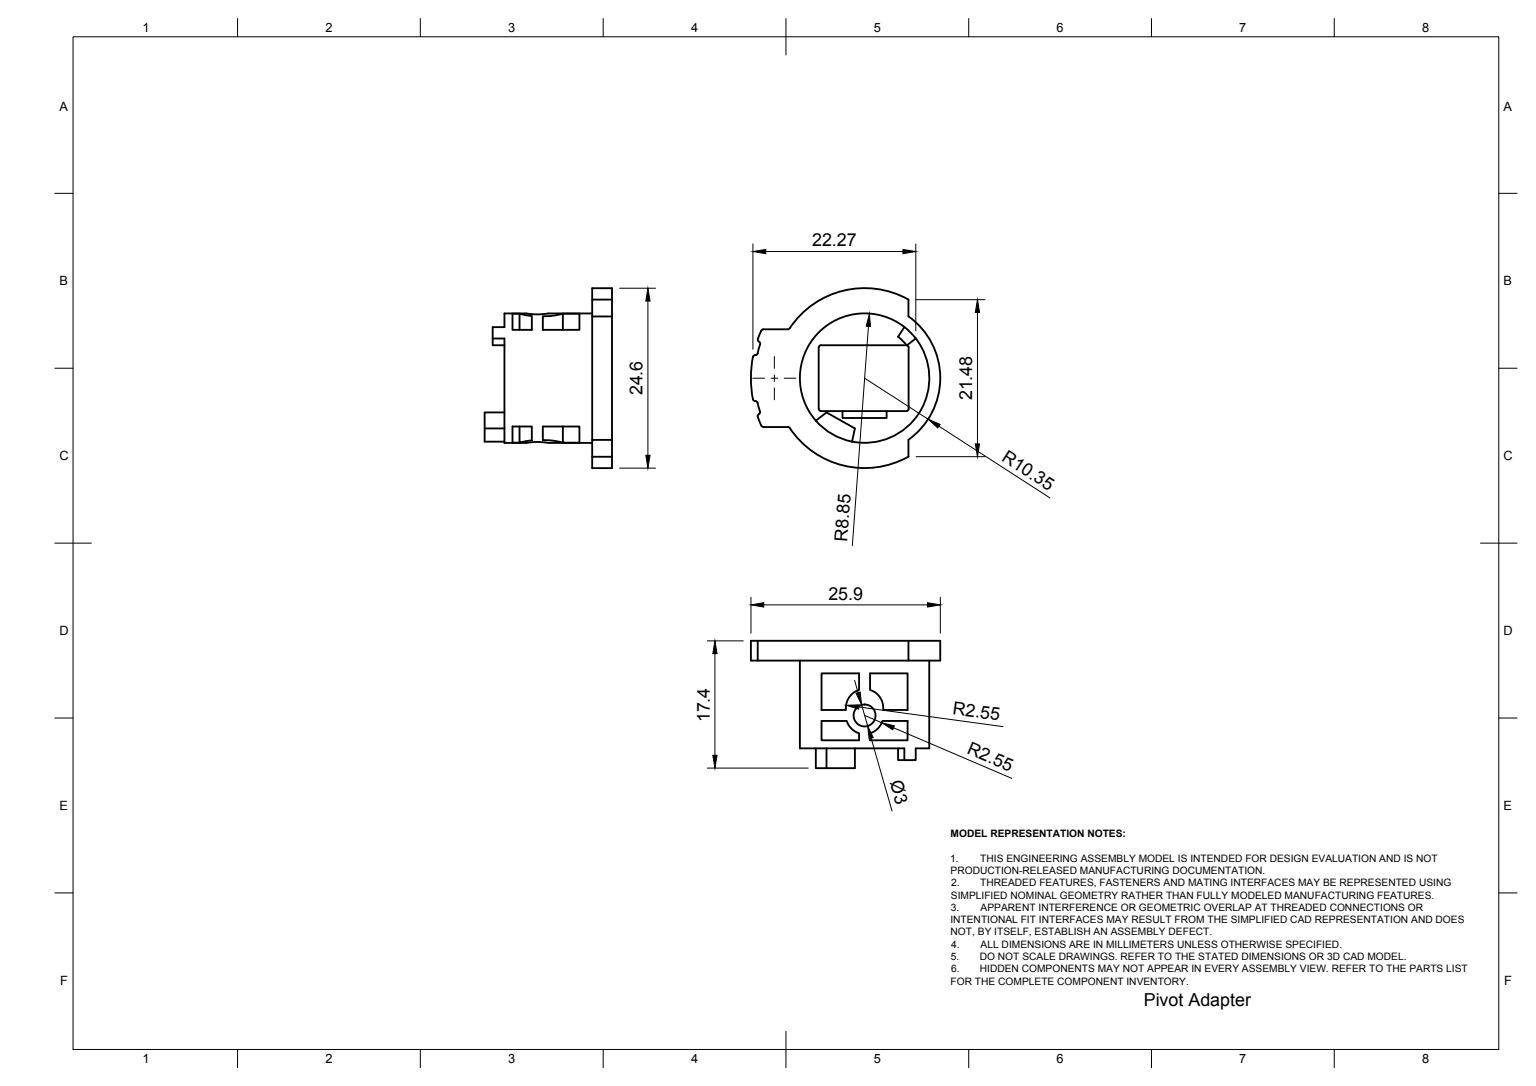
ISO-10303-21;
HEADER;
/* Generated by software containing ST-Developer
 * from STEP Tools, Inc. (www.steptools.com) 
 */

FILE_DESCRIPTION(
/* description */ ('STEP AP214'),
/* implementation_level */ '2;1');

FILE_NAME(
/* name */ 'Pivot Adapter.step',
/* time_stamp */ '2026-10-06T00:19:40-07:00',
/* author */ (''),
/* organization */ (''),
/* preprocessor_version */ 'ST-DEVELOPER v20.2',
/* originating_system */ 'Autodesk Translation Framework v15.15.0.0',
/* authorisation */ '');

FILE_SCHEMA (('AUTOMOTIVE_DESIGN { 1 0 10303 214 3 1 1 }'));
ENDSEC;

DATA;
#10=MECHANICAL_DESIGN_GEOMETRIC_PRESENTATION_REPRESENTATION('',(#2072),#98302);
#443=TOROIDAL_SURFACE('',#38348,4.64715395326,0.3);
#444=TOROIDAL_SURFACE('',#38570,0.6,0.3);
#445=TOROIDAL_SURFACE('',#38577,0.6,0.3);
#446=TOROIDAL_SURFACE('',#38588,0.6,0.3);
#447=TOROIDAL_SURFACE('',#38591,4.47840533247,0.3);
#448=TOROIDAL_SURFACE('',#38598,0.6,0.3);
#859=SPHERICAL_SURFACE('',#38392,4.49);
#860=SPHERICAL_SURFACE('',#38586,0.3);
#861=SPHERICAL_SURFACE('',#38596,0.3);
#1252=B_SPLINE_SURFACE_WITH_KNOTS('',5,5,((#98145,#98146,#98147,#98148,
#98149,#98150),(#98151,#98152,#98153,#98154,#98155,#98156),(#98157,#98158,
#98159,#98160,#98161,#98162),(#98163,#98164,#98165,#98166,#98167,#98168),
(#98169,#98170,#98171,#98172,#98173,#98174),(#98175,#98176,#98177,#98178,
#98179,#98180)),.UNSPECIFIED.,.F.,.F.,.F.,(6,6),(6,6),(2.82953519577,3.40560970652),
(0.,0.3),.UNSPECIFIED.);
#1253=B_SPLINE_SURFACE_WITH_KNOTS('',5,5,((#98207,#98208,#98209,#98210,
#98211,#98212),(#98213,#98214,#98215,#98216,#98217,#98218),(#98219,#98220,
#98221,#98222,#98223,#98224),(#98225,#98226,#98227,#98228,#98229,#98230),
(#98231,#98232,#98233,#98234,#98235,#98236),(#98237,#98238,#98239,#98240,
#98241,#98242)),.UNSPECIFIED.,.F.,.F.,.F.,(6,6),(6,6),(4.13551351914,4.71167786523),
(0.,0.3),.UNSPECIFIED.);
#1316=FACE_BOUND('',#7509,.T.);
#1317=FACE_BOUND('',#7564,.T.);
#1318=FACE_BOUND('',#7565,.T.);
#1319=FACE_BOUND('',#7599,.T.);
#1320=FACE_BOUND('',#7600,.T.);
#1321=FACE_BOUND('',#7601,.T.);
#1322=FACE_BOUND('',#7602,.T.);
#1323=FACE_BOUND('',#7603,.T.);
#1324=FACE_BOUND('',#7604,.T.);
#1325=FACE_BOUND('',#7605,.T.);
#1326=FACE_BOUND('',#7606,.T.);
#1327=FACE_BOUND('',#7607,.T.);
#1328=FACE_BOUND('',#7608,.T.);
#1329=FACE_BOUND('',#7619,.T.);
#1330=FACE_BOUND('',#7631,.T.);
#1331=FACE_BOUND('',#7634,.T.);
#2027=B_SPLINE_CURVE_WITH_KNOTS('',3,(#97465,#97466,#97467,#97468,#97469,
#97470,#97471),.UNSPECIFIED.,.F.,.F.,(4,3,4),(-4.71167786523,-4.28310422559678,
-4.13551354843282),.UNSPECIFIED.);
#2028=B_SPLINE_CURVE_WITH_KNOTS('',5,(#97472,#97473,#97474,#97475,#97476,
#97477),.UNSPECIFIED.,.F.,.F.,(6,6),(-3.40560970652,-2.82953519577),
 .UNSPECIFIED.);
#2029=B_SPLINE_CURVE_WITH_KNOTS('',3,(#97520,#97521,#97522,#97523,#97524,
#97525,#97526,#97527,#97528,#97529,#97530,#97531,#97532,#97533),
 .UNSPECIFIED.,.F.,.F.,(4,2,2,2,2,2,4),(0.22648251624436,0.28310233584346,
0.33972215544256,0.39634359396564,0.452965032488721,0.509586471011801,0.566207909534882),
 .UNSPECIFIED.);
#2030=B_SPLINE_CURVE_WITH_KNOTS('',3,(#97534,#97535,#97536,#97537,#97538,
#97539,#97540,#97541,#97542,#97543,#97544,#97545,#97546,#97547,#97548,#97549,
#97550,#97551,#97552,#97553,#97554,#97555,#97556),.UNSPECIFIED.,.F.,.F.,
(4,2,2,2,2,2,3,2,2,2,4),(0.566207909534882,0.622827729133982,0.679447548733081,
0.736067368332181,0.792687187931281,0.849308626454361,0.905930064977442,
0.962551503500522,1.0191729420236,1.0757927616227,1.1324125812218),
 .UNSPECIFIED.);
#2031=B_SPLINE_CURVE_WITH_KNOTS('',3,(#97583,#97584,#97585,#97586,#97587,
#97588,#97589,#97590,#97591,#97592),.UNSPECIFIED.,.F.,.F.,(4,2,2,2,4),(1.23339450152361,
1.25641237692672,1.35304825225328,1.44970846052674,1.5463686688002),
 .UNSPECIFIED.);
#2032=B_SPLINE_CURVE_WITH_KNOTS('',3,(#97622,#97623,#97624,#97625,#97626,
#97627,#97628,#97629,#97630,#97631),.UNSPECIFIED.,.F.,.F.,(4,2,2,2,4),(0.0736329241578598,
0.0966612073704035,0.193322414740807,0.289959287879085,0.312978165630601),
 .UNSPECIFIED.);
#2033=B_SPLINE_CURVE_WITH_KNOTS('',3,(#97652,#97653,#97654,#97655,#97656,
#97657,#97658,#97659,#97660,#97661),.UNSPECIFIED.,.F.,.F.,(4,2,2,2,4),(-0.699559397876643,
-0.676531114664321,-0.579869907293917,-0.48323303415564,-0.460214156403763),
 .UNSPECIFIED.);
#2034=B_SPLINE_CURVE_WITH_KNOTS('',3,(#97691,#97692,#97693,#97694,#97695,
#97696,#97697,#97698,#97699,#97700),.UNSPECIFIED.,.F.,.F.,(4,2,2,2,4),(0.773184334400102,
0.869844542673565,0.966504750947028,1.06314062627359,1.08615850163623),
 .UNSPECIFIED.);
#2035=B_SPLINE_CURVE_WITH_KNOTS('',3,(#97759,#97760,#97761,#97762,#97763,
#97764),.UNSPECIFIED.,.F.,.F.,(4,2,4),(0.566207909534882,0.622827729133982,
0.679447548733081),.UNSPECIFIED.);
#2036=B_SPLINE_CURVE_WITH_KNOTS('',3,(#97765,#97766,#97767,#97768,#97769,
#97770,#97771,#97772,#97773,#97774,#97775,#97776,#97777,#97778,#97779,#97780,
#97781,#97782,#97783,#97784,#97785,#97786,#97787,#97788,#97789,#97790,#97791,
#97792,#97793,#97794,#97795),.UNSPECIFIED.,.F.,.F.,(4,2,2,2,3,2,2,2,2,2,
2,2,2,2,4),(-0.22648251624436,-0.169862696645261,-0.113242877046161,-0.0566214385230804,
0.,0.0566214385230803,0.113242877046161,0.169862696645261,0.22648251624436,
0.28310233584346,0.33972215544256,0.39634359396564,0.452965032488721,0.509586471011801,
0.566207909534882),.UNSPECIFIED.);
#2037=B_SPLINE_CURVE_WITH_KNOTS('',3,(#97811,#97812,#97813,#97814,#97815,
#97816,#97817,#97818,#97819,#97820),.UNSPECIFIED.,.F.,.F.,(4,2,2,2,4),(-0.312974167276592,
-0.289956291873489,-0.193320416546926,-0.0966602082734631,0.),
 .UNSPECIFIED.);
#2038=B_SPLINE_CURVE_WITH_KNOTS('',3,(#97841,#97842,#97843,#97844,#97845,
#97846,#97847,#97848,#97849,#97850),.UNSPECIFIED.,.F.,.F.,(4,2,2,2,4),(-0.773184334400102,
-0.676524126126639,-0.579863917853176,-0.483228042526613,-0.460210167163969),
 .UNSPECIFIED.);
#2039=B_SPLINE_CURVE_WITH_KNOTS('',3,(#97873,#97874,#97875,#97876,#97877,
#97878,#97879,#97880,#97881,#97882),.UNSPECIFIED.,.F.,.F.,(4,2,2,2,4),(0.846825246192806,
0.869853529405128,0.966514736775532,1.06315160991381,1.08617048766569),
 .UNSPECIFIED.);
#2040=B_SPLINE_CURVE_WITH_KNOTS('',3,(#97903,#97904,#97905,#97906,#97907,
#97908,#97909,#97910,#97911,#97912),.UNSPECIFIED.,.F.,.F.,(4,2,2,2,4),(-1.47275171991159,
-1.44972343669905,-1.35306222932864,-1.25642535619036,-1.23340647843885),
 .UNSPECIFIED.);
#2041=B_SPLINE_CURVE_WITH_KNOTS('',3,(#98184,#98185,#98186,#98187,#98188,
#98189,#98190,#98191,#98192,#98193),.UNSPECIFIED.,.F.,.F.,(4,3,3,4),(-3.40560970652,
-3.15933845109684,-2.86373280280867,-2.82953519577),.UNSPECIFIED.);
#2042=B_SPLINE_CURVE_WITH_KNOTS('',3,(#98244,#98245,#98246,#98247,#98248,
#98249,#98250),.UNSPECIFIED.,.F.,.F.,(4,3,4),(-4.71167786523,-4.23171687797706,
-4.13551351914),.UNSPECIFIED.);
#2052=SHAPE_REPRESENTATION_RELATIONSHIP('SRR','None',#98349,#2062);
#2062=ADVANCED_BREP_SHAPE_REPRESENTATION('',(#2081),#98301);
#2072=STYLED_ITEM('',(#98399),#2081);
#2081=MANIFOLD_SOLID_BREP('Body1',#34178);
#2452=PLANE('',#38355);
#2453=PLANE('',#38358);
#2454=PLANE('',#38359);
#2455=PLANE('',#38362);
#2456=PLANE('',#38363);
#2457=PLANE('',#38365);
#2458=PLANE('',#38366);
#2459=PLANE('',#38367);
#2460=PLANE('',#38368);
#2461=PLANE('',#38372);
#2462=PLANE('',#38394);
#2463=PLANE('',#38402);
#2464=PLANE('',#38405);
#2465=PLANE('',#38407);
#2466=PLANE('',#38409);
#2467=PLANE('',#38411);
#2468=PLANE('',#38412);
#2469=PLANE('',#38414);
#2470=PLANE('',#38416);
#2471=PLANE('',#38418);
#2472=PLANE('',#38420);
#2473=PLANE('',#38422);
#2474=PLANE('',#38424);
#2475=PLANE('',#38427);
#2476=PLANE('',#38428);
#2477=PLANE('',#38430);
#2478=PLANE('',#38432);
#2479=PLANE('',#38434);
#2480=PLANE('',#38436);
#2481=PLANE('',#38437);
#2482=PLANE('',#38439);
#2483=PLANE('',#38441);
#2484=PLANE('',#38445);
#2485=PLANE('',#38449);
#2486=PLANE('',#38450);
#2487=PLANE('',#38455);
#2488=PLANE('',#38460);
#2489=PLANE('',#38462);
#2490=PLANE('',#38465);
#2491=PLANE('',#38466);
#2492=PLANE('',#38469);
#2493=PLANE('',#38470);
#2494=PLANE('',#38472);
#2495=PLANE('',#38476);
#2496=PLANE('',#38477);
#2497=PLANE('',#38481);
#2498=PLANE('',#38485);
#2499=PLANE('',#38512);
#2500=PLANE('',#38515);
#2501=PLANE('',#38520);
#2502=PLANE('',#38533);
#2503=PLANE('',#38540);
#2504=PLANE('',#38553);
#2505=PLANE('',#38556);
#2506=PLANE('',#38558);
#2507=PLANE('',#38559);
#2508=PLANE('',#38560);
#2509=PLANE('',#38562);
#2510=PLANE('',#38564);
#2511=PLANE('',#38568);
#2512=PLANE('',#38569);
#2513=PLANE('',#38576);
#2514=PLANE('',#38583);
#2515=PLANE('',#38594);
#2516=PLANE('',#38601);
#2517=PLANE('',#38602);
#2518=PLANE('',#38603);
#2519=PLANE('',#38604);
#2520=PLANE('',#38605);
#3234=CYLINDRICAL_SURFACE('',#38360,7.28184557105);
#3235=CYLINDRICAL_SURFACE('',#38370,1.2046272227);
#3236=CYLINDRICAL_SURFACE('',#38403,1.5);
#3237=CYLINDRICAL_SURFACE('',#38410,2.54997399005);
#3238=CYLINDRICAL_SURFACE('',#38419,2.55);
#3239=CYLINDRICAL_SURFACE('',#38426,2.55);
#3240=CYLINDRICAL_SURFACE('',#38435,2.54997399005);
#3241=CYLINDRICAL_SURFACE('',#38443,7.35);
#3242=CYLINDRICAL_SURFACE('',#38444,7.35);
#3243=CYLINDRICAL_SURFACE('',#38451,8.85);
#3244=CYLINDRICAL_SURFACE('',#38453,1.8);
#3245=CYLINDRICAL_SURFACE('',#38456,1.8);
#3246=CYLINDRICAL_SURFACE('',#38458,1.5);
#3247=CYLINDRICAL_SURFACE('',#38463,2.54997399005);
#3248=CYLINDRICAL_SURFACE('',#38467,2.54997399005);
#3249=CYLINDRICAL_SURFACE('',#38474,2.55);
#3250=CYLINDRICAL_SURFACE('',#38479,2.55);
#3251=CYLINDRICAL_SURFACE('',#38482,0.3);
#3252=CYLINDRICAL_SURFACE('',#38510,12.3);
#3253=CYLINDRICAL_SURFACE('',#38513,10.35);
#3254=CYLINDRICAL_SURFACE('',#38516,12.3);
#3255=CYLINDRICAL_SURFACE('',#38518,0.3);
#3256=CYLINDRICAL_SURFACE('',#38521,0.3);
#3257=CYLINDRICAL_SURFACE('',#38523,15.55);
#3258=CYLINDRICAL_SURFACE('',#38525,0.3);
#3259=CYLINDRICAL_SURFACE('',#38527,0.299999999999999);
#3260=CYLINDRICAL_SURFACE('',#38529,15.0204936174);
#3261=CYLINDRICAL_SURFACE('',#38531,0.3);
#3262=CYLINDRICAL_SURFACE('',#38534,0.3);
#3263=CYLINDRICAL_SURFACE('',#38536,15.55);
#3264=CYLINDRICAL_SURFACE('',#38538,0.3);
#3265=CYLINDRICAL_SURFACE('',#38541,0.3);
#3266=CYLINDRICAL_SURFACE('',#38543,15.0204936174);
#3267=CYLINDRICAL_SURFACE('',#38545,0.3);
#3268=CYLINDRICAL_SURFACE('',#38547,0.3);
#3269=CYLINDRICAL_SURFACE('',#38549,15.55);
#3270=CYLINDRICAL_SURFACE('',#38551,0.3);
#3271=CYLINDRICAL_SURFACE('',#38554,0.3);
#3272=CYLINDRICAL_SURFACE('',#38565,8.85);
#3273=CYLINDRICAL_SURFACE('',#38573,0.3);
#3274=CYLINDRICAL_SURFACE('',#38574,0.3);
#3275=CYLINDRICAL_SURFACE('',#38580,0.3);
#3276=CYLINDRICAL_SURFACE('',#38581,0.300000000000002);
#3277=CYLINDRICAL_SURFACE('',#38590,0.3);
#3278=CYLINDRICAL_SURFACE('',#38600,0.3);
#5294=FACE_OUTER_BOUND('',#7496,.T.);
#5295=FACE_OUTER_BOUND('',#7497,.T.);
#5296=FACE_OUTER_BOUND('',#7498,.T.);
#5297=FACE_OUTER_BOUND('',#7499,.T.);
#5298=FACE_OUTER_BOUND('',#7500,.T.);
#5299=FACE_OUTER_BOUND('',#7501,.T.);
#5300=FACE_OUTER_BOUND('',#7502,.T.);
#5301=FACE_OUTER_BOUND('',#7503,.T.);
#5302=FACE_OUTER_BOUND('',#7504,.T.);
#5303=FACE_OUTER_BOUND('',#7505,.T.);
#5304=FACE_OUTER_BOUND('',#7506,.T.);
#5305=FACE_OUTER_BOUND('',#7507,.T.);
#5306=FACE_OUTER_BOUND('',#7508,.T.);
#5307=FACE_OUTER_BOUND('',#7510,.T.);
#5308=FACE_OUTER_BOUND('',#7511,.T.);
#5309=FACE_OUTER_BOUND('',#7512,.T.);
#5310=FACE_OUTER_BOUND('',#7513,.T.);
#5311=FACE_OUTER_BOUND('',#7514,.T.);
#5312=FACE_OUTER_BOUND('',#7515,.T.);
#5313=FACE_OUTER_BOUND('',#7516,.T.);
#5314=FACE_OUTER_BOUND('',#7517,.T.);
#5315=FACE_OUTER_BOUND('',#7518,.T.);
#5316=FACE_OUTER_BOUND('',#7519,.T.);
#5317=FACE_OUTER_BOUND('',#7520,.T.);
#5318=FACE_OUTER_BOUND('',#7521,.T.);
#5319=FACE_OUTER_BOUND('',#7522,.T.);
#5320=FACE_OUTER_BOUND('',#7523,.T.);
#5321=FACE_OUTER_BOUND('',#7524,.T.);
#5322=FACE_OUTER_BOUND('',#7525,.T.);
#5323=FACE_OUTER_BOUND('',#7526,.T.);
#5324=FACE_OUTER_BOUND('',#7527,.T.);
#5325=FACE_OUTER_BOUND('',#7528,.T.);
#5326=FACE_OUTER_BOUND('',#7529,.T.);
#5327=FACE_OUTER_BOUND('',#7530,.T.);
#5328=FACE_OUTER_BOUND('',#7531,.T.);
#5329=FACE_OUTER_BOUND('',#7532,.T.);
#5330=FACE_OUTER_BOUND('',#7533,.T.);
#5331=FACE_OUTER_BOUND('',#7534,.T.);
#5332=FACE_OUTER_BOUND('',#7535,.T.);
#5333=FACE_OUTER_BOUND('',#7536,.T.);
#5334=FACE_OUTER_BOUND('',#7537,.T.);
#5335=FACE_OUTER_BOUND('',#7538,.T.);
#5336=FACE_OUTER_BOUND('',#7539,.T.);
#5337=FACE_OUTER_BOUND('',#7540,.T.);
#5338=FACE_OUTER_BOUND('',#7541,.T.);
#5339=FACE_OUTER_BOUND('',#7542,.T.);
#5340=FACE_OUTER_BOUND('',#7543,.T.);
#5341=FACE_OUTER_BOUND('',#7544,.T.);
#5342=FACE_OUTER_BOUND('',#7545,.T.);
#5343=FACE_OUTER_BOUND('',#7546,.T.);
#5344=FACE_OUTER_BOUND('',#7547,.T.);
#5345=FACE_OUTER_BOUND('',#7548,.T.);
#5346=FACE_OUTER_BOUND('',#7549,.T.);
#5347=FACE_OUTER_BOUND('',#7550,.T.);
#5348=FACE_OUTER_BOUND('',#7551,.T.);
#5349=FACE_OUTER_BOUND('',#7552,.T.);
#5350=FACE_OUTER_BOUND('',#7553,.T.);
#5351=FACE_OUTER_BOUND('',#7554,.T.);
#5352=FACE_OUTER_BOUND('',#7555,.T.);
#5353=FACE_OUTER_BOUND('',#7556,.T.);
#5354=FACE_OUTER_BOUND('',#7557,.T.);
#5355=FACE_OUTER_BOUND('',#7558,.T.);
#5356=FACE_OUTER_BOUND('',#7559,.T.);
#5357=FACE_OUTER_BOUND('',#7560,.T.);
#5358=FACE_OUTER_BOUND('',#7561,.T.);
#5359=FACE_OUTER_BOUND('',#7562,.T.);
#5360=FACE_OUTER_BOUND('',#7563,.T.);
#5361=FACE_OUTER_BOUND('',#7566,.T.);
#5362=FACE_OUTER_BOUND('',#7567,.T.);
#5363=FACE_OUTER_BOUND('',#7568,.T.);
#5364=FACE_OUTER_BOUND('',#7569,.T.);
#5365=FACE_OUTER_BOUND('',#7570,.T.);
#5366=FACE_OUTER_BOUND('',#7571,.T.);
#5367=FACE_OUTER_BOUND('',#7572,.T.);
#5368=FACE_OUTER_BOUND('',#7573,.T.);
#5369=FACE_OUTER_BOUND('',#7574,.T.);
#5370=FACE_OUTER_BOUND('',#7575,.T.);
#5371=FACE_OUTER_BOUND('',#7576,.T.);
#5372=FACE_OUTER_BOUND('',#7577,.T.);
#5373=FACE_OUTER_BOUND('',#7578,.T.);
#5374=FACE_OUTER_BOUND('',#7579,.T.);
#5375=FACE_OUTER_BOUND('',#7580,.T.);
#5376=FACE_OUTER_BOUND('',#7581,.T.);
#5377=FACE_OUTER_BOUND('',#7582,.T.);
#5378=FACE_OUTER_BOUND('',#7583,.T.);
#5379=FACE_OUTER_BOUND('',#7584,.T.);
#5380=FACE_OUTER_BOUND('',#7585,.T.);
#5381=FACE_OUTER_BOUND('',#7586,.T.);
#5382=FACE_OUTER_BOUND('',#7587,.T.);
#5383=FACE_OUTER_BOUND('',#7588,.T.);
#5384=FACE_OUTER_BOUND('',#7589,.T.);
#5385=FACE_OUTER_BOUND('',#7590,.T.);
#5386=FACE_OUTER_BOUND('',#7591,.T.);
#5387=FACE_OUTER_BOUND('',#7592,.T.);
#5388=FACE_OUTER_BOUND('',#7593,.T.);
#5389=FACE_OUTER_BOUND('',#7594,.T.);
#5390=FACE_OUTER_BOUND('',#7595,.T.);
#5391=FACE_OUTER_BOUND('',#7596,.T.);
#5392=FACE_OUTER_BOUND('',#7597,.T.);
#5393=FACE_OUTER_BOUND('',#7598,.T.);
#5394=FACE_OUTER_BOUND('',#7609,.T.);
#5395=FACE_OUTER_BOUND('',#7610,.T.);
#5396=FACE_OUTER_BOUND('',#7611,.T.);
#5397=FACE_OUTER_BOUND('',#7612,.T.);
#5398=FACE_OUTER_BOUND('',#7613,.T.);
#5399=FACE_OUTER_BOUND('',#7614,.T.);
#5400=FACE_OUTER_BOUND('',#7615,.T.);
#5401=FACE_OUTER_BOUND('',#7616,.T.);
#5402=FACE_OUTER_BOUND('',#7617,.T.);
#5403=FACE_OUTER_BOUND('',#7618,.T.);
#5404=FACE_OUTER_BOUND('',#7620,.T.);
#5405=FACE_OUTER_BOUND('',#7621,.T.);
#5406=FACE_OUTER_BOUND('',#7622,.T.);
#5407=FACE_OUTER_BOUND('',#7623,.T.);
#5408=FACE_OUTER_BOUND('',#7624,.T.);
#5409=FACE_OUTER_BOUND('',#7625,.T.);
#5410=FACE_OUTER_BOUND('',#7626,.T.);
#5411=FACE_OUTER_BOUND('',#7627,.T.);
#5412=FACE_OUTER_BOUND('',#7628,.T.);
#5413=FACE_OUTER_BOUND('',#7629,.T.);
#5414=FACE_OUTER_BOUND('',#7630,.T.);
#5415=FACE_OUTER_BOUND('',#7632,.T.);
#5416=FACE_OUTER_BOUND('',#7633,.T.);
#5417=FACE_OUTER_BOUND('',#7635,.T.);
#5418=FACE_OUTER_BOUND('',#7636,.T.);
#7496=EDGE_LOOP('',(#31335,#31336,#31337,#31338,#31339,#31340));
#7497=EDGE_LOOP('',(#31341,#31342,#31343,#31344,#31345));
#7498=EDGE_LOOP('',(#31346,#31347,#31348,#31349));
#7499=EDGE_LOOP('',(#31350,#31351,#31352,#31353));
#7500=EDGE_LOOP('',(#31354,#31355,#31356,#31357));
#7501=EDGE_LOOP('',(#31358,#31359,#31360,#31361));
#7502=EDGE_LOOP('',(#31362,#31363,#31364,#31365));
#7503=EDGE_LOOP('',(#31366,#31367,#31368,#31369));
#7504=EDGE_LOOP('',(#31370,#31371,#31372,#31373));
#7505=EDGE_LOOP('',(#31374,#31375,#31376,#31377));
#7506=EDGE_LOOP('',(#31378));
#7507=EDGE_LOOP('',(#31379,#31380,#31381,#31382));
#7508=EDGE_LOOP('',(#31383,#31384,#31385,#31386,#31387,#31388,#31389,#31390,
#31391,#31392,#31393,#31394,#31395,#31396,#31397,#31398,#31399,#31400,#31401,
#31402,#31403,#31404,#31405,#31406,#31407,#31408,#31409,#31410,#31411,#31412));
#7509=EDGE_LOOP('',(#31413));
#7510=EDGE_LOOP('',(#31414,#31415,#31416,#31417));
#7511=EDGE_LOOP('',(#31418,#31419,#31420,#31421,#31422,#31423,#31424,#31425,
#31426,#31427,#31428,#31429,#31430,#31431,#31432,#31433,#31434,#31435,#31436,
#31437,#31438,#31439));
#7512=EDGE_LOOP('',(#31440,#31441,#31442,#31443,#31444,#31445,#31446,#31447));
#7513=EDGE_LOOP('',(#31448,#31449,#31450,#31451,#31452));
#7514=EDGE_LOOP('',(#31453,#31454,#31455,#31456,#31457,#31458));
#7515=EDGE_LOOP('',(#31459,#31460,#31461));
#7516=EDGE_LOOP('',(#31462,#31463,#31464,#31465));
#7517=EDGE_LOOP('',(#31466,#31467,#31468,#31469));
#7518=EDGE_LOOP('',(#31470,#31471,#31472,#31473));
#7519=EDGE_LOOP('',(#31474,#31475,#31476));
#7520=EDGE_LOOP('',(#31477,#31478,#31479));
#7521=EDGE_LOOP('',(#31480,#31481,#31482,#31483,#31484));
#7522=EDGE_LOOP('',(#31485,#31486,#31487,#31488));
#7523=EDGE_LOOP('',(#31489,#31490,#31491,#31492));
#7524=EDGE_LOOP('',(#31493,#31494,#31495));
#7525=EDGE_LOOP('',(#31496,#31497,#31498,#31499,#31500));
#7526=EDGE_LOOP('',(#31501,#31502,#31503));
#7527=EDGE_LOOP('',(#31504,#31505,#31506,#31507));
#7528=EDGE_LOOP('',(#31508,#31509,#31510,#31511));
#7529=EDGE_LOOP('',(#31512,#31513,#31514));
#7530=EDGE_LOOP('',(#31515,#31516,#31517));
#7531=EDGE_LOOP('',(#31518,#31519,#31520,#31521,#31522,#31523));
#7532=EDGE_LOOP('',(#31524,#31525,#31526,#31527));
#7533=EDGE_LOOP('',(#31528,#31529,#31530,#31531));
#7534=EDGE_LOOP('',(#31532,#31533,#31534,#31535));
#7535=EDGE_LOOP('',(#31536,#31537,#31538));
#7536=EDGE_LOOP('',(#31539,#31540));
#7537=EDGE_LOOP('',(#31541,#31542));
#7538=EDGE_LOOP('',(#31543,#31544,#31545,#31546));
#7539=EDGE_LOOP('',(#31547,#31548,#31549,#31550));
#7540=EDGE_LOOP('',(#31551,#31552,#31553,#31554));
#7541=EDGE_LOOP('',(#31555,#31556,#31557,#31558));
#7542=EDGE_LOOP('',(#31559,#31560,#31561,#31562));
#7543=EDGE_LOOP('',(#31563,#31564,#31565,#31566));
#7544=EDGE_LOOP('',(#31567,#31568,#31569,#31570));
#7545=EDGE_LOOP('',(#31571,#31572,#31573,#31574));
#7546=EDGE_LOOP('',(#31575,#31576,#31577,#31578));
#7547=EDGE_LOOP('',(#31579,#31580,#31581,#31582,#31583));
#7548=EDGE_LOOP('',(#31584,#31585,#31586));
#7549=EDGE_LOOP('',(#31587,#31588,#31589,#31590));
#7550=EDGE_LOOP('',(#31591,#31592,#31593,#31594));
#7551=EDGE_LOOP('',(#31595,#31596,#31597,#31598));
#7552=EDGE_LOOP('',(#31599,#31600,#31601,#31602));
#7553=EDGE_LOOP('',(#31603,#31604,#31605,#31606));
#7554=EDGE_LOOP('',(#31607,#31608,#31609,#31610));
#7555=EDGE_LOOP('',(#31611,#31612,#31613));
#7556=EDGE_LOOP('',(#31614,#31615,#31616));
#7557=EDGE_LOOP('',(#31617,#31618,#31619,#31620));
#7558=EDGE_LOOP('',(#31621,#31622,#31623,#31624));
#7559=EDGE_LOOP('',(#31625,#31626,#31627));
#7560=EDGE_LOOP('',(#31628,#31629,#31630,#31631));
#7561=EDGE_LOOP('',(#31632,#31633,#31634,#31635));
#7562=EDGE_LOOP('',(#31636,#31637,#31638,#31639));
#7563=EDGE_LOOP('',(#31640,#31641,#31642,#31643,#31644,#31645,#31646,#31647,
#31648,#31649,#31650,#31651,#31652,#31653,#31654,#31655,#31656,#31657,#31658,
#31659,#31660,#31661,#31662,#31663,#31664,#31665));
#7564=EDGE_LOOP('',(#31666,#31667,#31668,#31669));
#7565=EDGE_LOOP('',(#31670,#31671,#31672,#31673,#31674,#31675,#31676,#31677,
#31678,#31679,#31680,#31681,#31682,#31683,#31684,#31685,#31686,#31687,#31688,
#31689,#31690,#31691,#31692,#31693,#31694,#31695,#31696,#31697,#31698,#31699,
#31700,#31701,#31702,#31703,#31704,#31705,#31706,#31707));
#7566=EDGE_LOOP('',(#31708,#31709,#31710,#31711));
#7567=EDGE_LOOP('',(#31712,#31713,#31714,#31715));
#7568=EDGE_LOOP('',(#31716,#31717,#31718,#31719));
#7569=EDGE_LOOP('',(#31720,#31721,#31722,#31723));
#7570=EDGE_LOOP('',(#31724,#31725,#31726,#31727));
#7571=EDGE_LOOP('',(#31728,#31729,#31730,#31731));
#7572=EDGE_LOOP('',(#31732,#31733,#31734,#31735));
#7573=EDGE_LOOP('',(#31736,#31737,#31738,#31739));
#7574=EDGE_LOOP('',(#31740,#31741,#31742,#31743));
#7575=EDGE_LOOP('',(#31744,#31745,#31746,#31747));
#7576=EDGE_LOOP('',(#31748,#31749,#31750,#31751));
#7577=EDGE_LOOP('',(#31752,#31753,#31754,#31755));
#7578=EDGE_LOOP('',(#31756,#31757,#31758,#31759));
#7579=EDGE_LOOP('',(#31760,#31761,#31762,#31763));
#7580=EDGE_LOOP('',(#31764,#31765,#31766,#31767));
#7581=EDGE_LOOP('',(#31768,#31769,#31770,#31771));
#7582=EDGE_LOOP('',(#31772,#31773,#31774,#31775));
#7583=EDGE_LOOP('',(#31776,#31777,#31778,#31779));
#7584=EDGE_LOOP('',(#31780,#31781,#31782,#31783));
#7585=EDGE_LOOP('',(#31784,#31785,#31786,#31787));
#7586=EDGE_LOOP('',(#31788,#31789,#31790,#31791));
#7587=EDGE_LOOP('',(#31792,#31793,#31794,#31795));
#7588=EDGE_LOOP('',(#31796,#31797,#31798,#31799));
#7589=EDGE_LOOP('',(#31800,#31801,#31802,#31803));
#7590=EDGE_LOOP('',(#31804,#31805,#31806,#31807));
#7591=EDGE_LOOP('',(#31808,#31809,#31810,#31811));
#7592=EDGE_LOOP('',(#31812,#31813,#31814));
#7593=EDGE_LOOP('',(#31815,#31816,#31817,#31818,#31819));
#7594=EDGE_LOOP('',(#31820,#31821,#31822,#31823,#31824,#31825));
#7595=EDGE_LOOP('',(#31826,#31827,#31828));
#7596=EDGE_LOOP('',(#31829,#31830,#31831));
#7597=EDGE_LOOP('',(#31832,#31833,#31834,#31835,#31836,#31837));
#7598=EDGE_LOOP('',(#31838,#31839,#31840,#31841,#31842,#31843,#31844,#31845,
#31846,#31847,#31848,#31849));
#7599=EDGE_LOOP('',(#31850,#31851,#31852,#31853,#31854));
#7600=EDGE_LOOP('',(#31855,#31856,#31857,#31858,#31859));
#7601=EDGE_LOOP('',(#31860,#31861,#31862,#31863,#31864,#31865));
#7602=EDGE_LOOP('',(#31866,#31867));
#7603=EDGE_LOOP('',(#31868,#31869,#31870,#31871,#31872,#31873));
#7604=EDGE_LOOP('',(#31874,#31875,#31876,#31877,#31878));
#7605=EDGE_LOOP('',(#31879,#31880,#31881,#31882,#31883));
#7606=EDGE_LOOP('',(#31884,#31885,#31886,#31887,#31888,#31889));
#7607=EDGE_LOOP('',(#31890,#31891,#31892,#31893,#31894,#31895));
#7608=EDGE_LOOP('',(#31896,#31897));
#7609=EDGE_LOOP('',(#31898,#31899,#31900,#31901,#31902));
#7610=EDGE_LOOP('',(#31903,#31904,#31905));
#7611=EDGE_LOOP('',(#31906,#31907,#31908,#31909));
#7612=EDGE_LOOP('',(#31910,#31911,#31912,#31913));
#7613=EDGE_LOOP('',(#31914,#31915,#31916,#31917));
#7614=EDGE_LOOP('',(#31918,#31919,#31920,#31921));
#7615=EDGE_LOOP('',(#31922,#31923,#31924,#31925));
#7616=EDGE_LOOP('',(#31926,#31927,#31928,#31929));
#7617=EDGE_LOOP('',(#31930,#31931,#31932,#31933));
#7618=EDGE_LOOP('',(#31934,#31935,#31936,#31937));
#7619=EDGE_LOOP('',(#31938));
#7620=EDGE_LOOP('',(#31939,#31940,#31941,#31942));
#7621=EDGE_LOOP('',(#31943,#31944,#31945));
#7622=EDGE_LOOP('',(#31946,#31947,#31948,#31949));
#7623=EDGE_LOOP('',(#31950,#31951,#31952,#31953,#31954));
#7624=EDGE_LOOP('',(#31955,#31956,#31957,#31958));
#7625=EDGE_LOOP('',(#31959,#31960,#31961,#31962));
#7626=EDGE_LOOP('',(#31963,#31964,#31965,#31966));
#7627=EDGE_LOOP('',(#31967,#31968,#31969));
#7628=EDGE_LOOP('',(#31970,#31971,#31972,#31973));
#7629=EDGE_LOOP('',(#31974,#31975,#31976,#31977,#31978));
#7630=EDGE_LOOP('',(#31979,#31980,#31981,#31982,#31983,#31984,#31985,#31986,
#31987,#31988,#31989,#31990,#31991,#31992,#31993,#31994,#31995,#31996,#31997,
#31998,#31999,#32000,#32001,#32002,#32003,#32004));
#7631=EDGE_LOOP('',(#32005));
#7632=EDGE_LOOP('',(#32006,#32007,#32008,#32009));
#7633=EDGE_LOOP('',(#32010,#32011,#32012,#32013));
#7634=EDGE_LOOP('',(#32014));
#7635=EDGE_LOOP('',(#32015,#32016,#32017,#32018));
#7636=EDGE_LOOP('',(#32019,#32020,#32021,#32022));
#9284=LINE('',#97349,#11124);
#9285=LINE('',#97353,#11125);
#9286=LINE('',#97354,#11126);
#9287=LINE('',#97357,#11127);
#9288=LINE('',#97359,#11128);
#9289=LINE('',#97360,#11129);
#9290=LINE('',#97363,#11130);
#9291=LINE('',#97364,#11131);
#9292=LINE('',#97367,#11132);
#9293=LINE('',#97371,#11133);
#9294=LINE('',#97372,#11134);
#9295=LINE('',#97376,#11135);
#9296=LINE('',#97378,#11136);
#9297=LINE('',#97381,#11137);
#9298=LINE('',#97385,#11138);
#9299=LINE('',#97386,#11139);
#9300=LINE('',#97387,#11140);
#9301=LINE('',#97390,#11141);
#9302=LINE('',#97391,#11142);
#9303=LINE('',#97394,#11143);
#9304=LINE('',#97395,#11144);
#9305=LINE('',#97401,#11145);
#9306=LINE('',#97405,#11146);
#9307=LINE('',#97409,#11147);
#9308=LINE('',#97413,#11148);
#9309=LINE('',#97419,#11149);
#9310=LINE('',#97425,#11150);
#9311=LINE('',#97441,#11151);
#9312=LINE('',#97447,#11152);
#9313=LINE('',#97453,#11153);
#9314=LINE('',#97457,#11154);
#9315=LINE('',#97460,#11155);
#9316=LINE('',#97482,#11156);
#9317=LINE('',#97486,#11157);
#9318=LINE('',#97488,#11158);
#9319=LINE('',#97490,#11159);
#9320=LINE('',#97492,#11160);
#9321=LINE('',#97494,#11161);
#9322=LINE('',#97498,#11162);
#9323=LINE('',#97501,#11163);
#9324=LINE('',#97509,#11164);
#9325=LINE('',#97510,#11165);
#9326=LINE('',#97512,#11166);
#9327=LINE('',#97514,#11167);
#9328=LINE('',#97515,#11168);
#9329=LINE('',#97516,#11169);
#9330=LINE('',#97558,#11170);
#9331=LINE('',#97563,#11171);
#9332=LINE('',#97565,#11172);
#9333=LINE('',#97567,#11173);
#9334=LINE('',#97571,#11174);
#9335=LINE('',#97572,#11175);
#9336=LINE('',#97575,#11176);
#9337=LINE('',#97579,#11177);
#9338=LINE('',#97580,#11178);
#9339=LINE('',#97593,#11179);
#9340=LINE('',#97596,#11180);
#9341=LINE('',#97597,#11181);
#9342=LINE('',#97605,#11182);
#9343=LINE('',#97606,#11183);
#9344=LINE('',#97609,#11184);
#9345=LINE('',#97611,#11185);
#9346=LINE('',#97614,#11186);
#9347=LINE('',#97617,#11187);
#9348=LINE('',#97618,#11188);
#9349=LINE('',#97621,#11189);
#9350=LINE('',#97637,#11190);
#9351=LINE('',#97639,#11191);
#9352=LINE('',#97641,#11192);
#9353=LINE('',#97644,#11193);
#9354=LINE('',#97648,#11194);
#9355=LINE('',#97651,#11195);
#9356=LINE('',#97664,#11196);
#9357=LINE('',#97665,#11197);
#9358=LINE('',#97673,#11198);
#9359=LINE('',#97674,#11199);
#9360=LINE('',#97677,#11200);
#9361=LINE('',#97679,#11201);
#9362=LINE('',#97681,#11202);
#9363=LINE('',#97684,#11203);
#9364=LINE('',#97687,#11204);
#9365=LINE('',#97688,#11205);
#9366=LINE('',#97701,#11206);
#9367=LINE('',#97704,#11207);
#9368=LINE('',#97705,#11208);
#9369=LINE('',#97712,#11209);
#9370=LINE('',#97717,#11210);
#9371=LINE('',#97719,#11211);
#9372=LINE('',#97720,#11212);
#9373=LINE('',#97722,#11213);
#9374=LINE('',#97723,#11214);
#9375=LINE('',#97731,#11215);
#9376=LINE('',#97734,#11216);
#9377=LINE('',#97736,#11217);
#9378=LINE('',#97741,#11218);
#9379=LINE('',#97742,#11219);
#9380=LINE('',#97746,#11220);
#9381=LINE('',#97749,#11221);
#9382=LINE('',#97750,#11222);
#9383=LINE('',#97757,#11223);
#9384=LINE('',#97801,#11224);
#9385=LINE('',#97802,#11225);
#9386=LINE('',#97805,#11226);
#9387=LINE('',#97807,#11227);
#9388=LINE('',#97808,#11228);
#9389=LINE('',#97822,#11229);
#9390=LINE('',#97827,#11230);
#9391=LINE('',#97828,#11231);
#9392=LINE('',#97829,#11232);
#9393=LINE('',#97833,#11233);
#9394=LINE('',#97835,#11234);
#9395=LINE('',#97837,#11235);
#9396=LINE('',#97838,#11236);
#9397=LINE('',#97852,#11237);
#9398=LINE('',#97856,#11238);
#9399=LINE('',#97858,#11239);
#9400=LINE('',#97859,#11240);
#9401=LINE('',#97863,#11241);
#9402=LINE('',#97867,#11242);
#9403=LINE('',#97870,#11243);
#9404=LINE('',#97884,#11244);
#9405=LINE('',#97888,#11245);
#9406=LINE('',#97890,#11246);
#9407=LINE('',#97891,#11247);
#9408=LINE('',#97895,#11248);
#9409=LINE('',#97897,#11249);
#9410=LINE('',#97902,#11250);
#9411=LINE('',#97916,#11251);
#9412=LINE('',#97918,#11252);
#9413=LINE('',#97919,#11253);
#9414=LINE('',#97925,#11254);
#9415=LINE('',#97929,#11255);
#9416=LINE('',#97935,#11256);
#9417=LINE('',#97949,#11257);
#9418=LINE('',#97957,#11258);
#9419=LINE('',#97971,#11259);
#9420=LINE('',#97977,#11260);
#9421=LINE('',#97983,#11261);
#9422=LINE('',#97987,#11262);
#9423=LINE('',#97991,#11263);
#9424=LINE('',#97993,#11264);
#9425=LINE('',#97997,#11265);
#9426=LINE('',#97998,#11266);
#9427=LINE('',#98002,#11267);
#9428=LINE('',#98005,#11268);
#9429=LINE('',#98006,#11269);
#9430=LINE('',#98009,#11270);
#9431=LINE('',#98013,#11271);
#9432=LINE('',#98017,#11272);
#9433=LINE('',#98018,#11273);
#9434=LINE('',#98022,#11274);
#9435=LINE('',#98026,#11275);
#9436=LINE('',#98030,#11276);
#9437=LINE('',#98033,#11277);
#9438=LINE('',#98037,#11278);
#9439=LINE('',#98041,#11279);
#9440=LINE('',#98045,#11280);
#9441=LINE('',#98046,#11281);
#9442=LINE('',#98050,#11282);
#9443=LINE('',#98053,#11283);
#9444=LINE('',#98058,#11284);
#9445=LINE('',#98061,#11285);
#9446=LINE('',#98062,#11286);
#9447=LINE('',#98065,#11287);
#9448=LINE('',#98069,#11288);
#9449=LINE('',#98073,#11289);
#9450=LINE('',#98078,#11290);
#9451=LINE('',#98081,#11291);
#9452=LINE('',#98086,#11292);
#9453=LINE('',#98089,#11293);
#9454=LINE('',#98090,#11294);
#9455=LINE('',#98096,#11295);
#9456=LINE('',#98098,#11296);
#9457=LINE('',#98101,#11297);
#9458=LINE('',#98102,#11298);
#9459=LINE('',#98108,#11299);
#9460=LINE('',#98110,#11300);
#9461=LINE('',#98113,#11301);
#9462=LINE('',#98117,#11302);
#9463=LINE('',#98119,#11303);
#9464=LINE('',#98126,#11304);
#9465=LINE('',#98129,#11305);
#9466=LINE('',#98132,#11306);
#9467=LINE('',#98138,#11307);
#9468=LINE('',#98141,#11308);
#9469=LINE('',#98144,#11309);
#9470=LINE('',#98200,#11310);
#9471=LINE('',#98206,#11311);
#9472=LINE('',#98260,#11312);
#9473=LINE('',#98261,#11313);
#9474=LINE('',#98264,#11314);
#9475=LINE('',#98265,#11315);
#9476=LINE('',#98267,#11316);
#11124=VECTOR('',#48397,1000.);
#11125=VECTOR('',#48400,1000.);
#11126=VECTOR('',#48401,1000.);
#11127=VECTOR('',#48404,1000.);
#11128=VECTOR('',#48405,1000.);
#11129=VECTOR('',#48406,1000.);
#11130=VECTOR('',#48409,1000.);
#11131=VECTOR('',#48410,1000.);
#11132=VECTOR('',#48413,1000.);
#11133=VECTOR('',#48418,1000.);
#11134=VECTOR('',#48419,1000.);
#11135=VECTOR('',#48422,1000.);
#11136=VECTOR('',#48423,1000.);
#11137=VECTOR('',#48426,1000.);
#11138=VECTOR('',#48429,1000.);
#11139=VECTOR('',#48430,1000.);
#11140=VECTOR('',#48431,1000.);
#11141=VECTOR('',#48434,1000.);
#11142=VECTOR('',#48435,1000.);
#11143=VECTOR('',#48438,1000.);
#11144=VECTOR('',#48439,1000.);
#11145=VECTOR('',#48446,1.2046272227);
#11146=VECTOR('',#48451,1000.);
#11147=VECTOR('',#48454,1000.);
#11148=VECTOR('',#48457,1000.);
#11149=VECTOR('',#48462,1000.);
#11150=VECTOR('',#48467,1000.);
#11151=VECTOR('',#48482,1000.);
#11152=VECTOR('',#48487,1000.);
#11153=VECTOR('',#48492,1000.);
#11154=VECTOR('',#48495,1000.);
#11155=VECTOR('',#48498,1000.);
#11156=VECTOR('',#48507,1000.);
#11157=VECTOR('',#48510,1000.);
#11158=VECTOR('',#48511,1000.);
#11159=VECTOR('',#48512,1000.);
#11160=VECTOR('',#48513,1000.);
#11161=VECTOR('',#48514,1000.);
#11162=VECTOR('',#48517,1000.);
#11163=VECTOR('',#48520,1000.);
#11164=VECTOR('',#48529,1000.);
#11165=VECTOR('',#48530,1000.);
#11166=VECTOR('',#48531,1000.);
#11167=VECTOR('',#48532,1000.);
#11168=VECTOR('',#48533,1000.);
#11169=VECTOR('',#48534,1000.);
#11170=VECTOR('',#48537,1.5);
#11171=VECTOR('',#48542,1000.);
#11172=VECTOR('',#48543,1000.);
#11173=VECTOR('',#48544,1000.);
#11174=VECTOR('',#48547,1000.);
#11175=VECTOR('',#48548,1000.);
#11176=VECTOR('',#48551,1000.);
#11177=VECTOR('',#48556,1000.);
#11178=VECTOR('',#48557,1000.);
#11179=VECTOR('',#48560,1000.);
#11180=VECTOR('',#48563,1000.);
#11181=VECTOR('',#48564,1000.);
#11182=VECTOR('',#48573,1000.);
#11183=VECTOR('',#48574,1000.);
#11184=VECTOR('',#48577,1000.);
#11185=VECTOR('',#48578,1000.);
#11186=VECTOR('',#48581,1000.);
#11187=VECTOR('',#48584,1000.);
#11188=VECTOR('',#48585,1000.);
#11189=VECTOR('',#48588,1000.);
#11190=VECTOR('',#48595,1000.);
#11191=VECTOR('',#48596,1000.);
#11192=VECTOR('',#48597,1000.);
#11193=VECTOR('',#48600,1000.);
#11194=VECTOR('',#48605,1000.);
#11195=VECTOR('',#48608,1000.);
#11196=VECTOR('',#48611,1000.);
#11197=VECTOR('',#48612,1000.);
#11198=VECTOR('',#48621,1000.);
#11199=VECTOR('',#48622,1000.);
#11200=VECTOR('',#48625,1000.);
#11201=VECTOR('',#48626,1000.);
#11202=VECTOR('',#48627,1000.);
#11203=VECTOR('',#48630,1000.);
#11204=VECTOR('',#48633,1000.);
#11205=VECTOR('',#48634,1000.);
#11206=VECTOR('',#48637,1000.);
#11207=VECTOR('',#48640,1000.);
#11208=VECTOR('',#48641,1000.);
#11209=VECTOR('',#48650,1000.);
#11210=VECTOR('',#48655,1000.);
#11211=VECTOR('',#48658,1000.);
#11212=VECTOR('',#48659,1000.);
#11213=VECTOR('',#48662,1000.);
#11214=VECTOR('',#48663,1000.);
#11215=VECTOR('',#48670,1000.);
#11216=VECTOR('',#48675,1000.);
#11217=VECTOR('',#48678,1000.);
#11218=VECTOR('',#48683,1000.);
#11219=VECTOR('',#48684,1000.);
#11220=VECTOR('',#48689,1000.);
#11221=VECTOR('',#48692,1000.);
#11222=VECTOR('',#48693,1000.);
#11223=VECTOR('',#48702,1.5);
#11224=VECTOR('',#48707,1000.);
#11225=VECTOR('',#48708,1000.);
#11226=VECTOR('',#48711,1000.);
#11227=VECTOR('',#48712,1000.);
#11228=VECTOR('',#48713,1000.);
#11229=VECTOR('',#48716,1000.);
#11230=VECTOR('',#48721,1000.);
#11231=VECTOR('',#48722,1000.);
#11232=VECTOR('',#48723,1000.);
#11233=VECTOR('',#48726,1000.);
#11234=VECTOR('',#48727,1000.);
#11235=VECTOR('',#48728,1000.);
#11236=VECTOR('',#48729,1000.);
#11237=VECTOR('',#48732,1000.);
#11238=VECTOR('',#48737,1000.);
#11239=VECTOR('',#48738,1000.);
#11240=VECTOR('',#48739,1000.);
#11241=VECTOR('',#48744,1000.);
#11242=VECTOR('',#48747,1000.);
#11243=VECTOR('',#48750,1000.);
#11244=VECTOR('',#48753,1000.);
#11245=VECTOR('',#48758,1000.);
#11246=VECTOR('',#48759,1000.);
#11247=VECTOR('',#48760,1000.);
#11248=VECTOR('',#48763,1000.);
#11249=VECTOR('',#48764,1000.);
#11250=VECTOR('',#48769,1000.);
#11251=VECTOR('',#48774,1000.);
#11252=VECTOR('',#48775,1000.);
#11253=VECTOR('',#48776,1000.);
#11254=VECTOR('',#48783,1000.);
#11255=VECTOR('',#48786,1000.);
#11256=VECTOR('',#48791,1000.);
#11257=VECTOR('',#48804,1000.);
#11258=VECTOR('',#48811,1000.);
#11259=VECTOR('',#48824,1000.);
#11260=VECTOR('',#48829,1000.);
#11261=VECTOR('',#48836,1000.);
#11262=VECTOR('',#48839,1000.);
#11263=VECTOR('',#48844,1000.);
#11264=VECTOR('',#48845,1000.);
#11265=VECTOR('',#48850,1000.);
#11266=VECTOR('',#48851,1000.);
#11267=VECTOR('',#48856,1000.);
#11268=VECTOR('',#48859,1000.);
#11269=VECTOR('',#48860,1000.);
#11270=VECTOR('',#48863,1000.);
#11271=VECTOR('',#48868,1000.);
#11272=VECTOR('',#48873,1000.);
#11273=VECTOR('',#48874,1000.);
#11274=VECTOR('',#48879,1000.);
#11275=VECTOR('',#48884,1000.);
#11276=VECTOR('',#48889,1000.);
#11277=VECTOR('',#48892,1000.);
#11278=VECTOR('',#48897,1000.);
#11279=VECTOR('',#48902,1000.);
#11280=VECTOR('',#48907,1000.);
#11281=VECTOR('',#48908,1000.);
#11282=VECTOR('',#48913,1000.);
#11283=VECTOR('',#48916,1000.);
#11284=VECTOR('',#48923,1000.);
#11285=VECTOR('',#48926,1000.);
#11286=VECTOR('',#48927,1000.);
#11287=VECTOR('',#48930,1000.);
#11288=VECTOR('',#48935,1000.);
#11289=VECTOR('',#48940,1000.);
#11290=VECTOR('',#48947,1000.);
#11291=VECTOR('',#48950,1000.);
#11292=VECTOR('',#48957,1000.);
#11293=VECTOR('',#48960,1000.);
#11294=VECTOR('',#48961,1000.);
#11295=VECTOR('',#48970,1000.);
#11296=VECTOR('',#48973,1000.);
#11297=VECTOR('',#48976,1000.);
#11298=VECTOR('',#48977,1000.);
#11299=VECTOR('',#48986,1000.);
#11300=VECTOR('',#48989,1000.);
#11301=VECTOR('',#48992,8.85);
#11302=VECTOR('',#48997,1000.);
#11303=VECTOR('',#49000,1000.);
#11304=VECTOR('',#49011,1000.);
#11305=VECTOR('',#49014,1000.);
#11306=VECTOR('',#49019,1000.);
#11307=VECTOR('',#49028,1000.);
#11308=VECTOR('',#49031,1000.);
#11309=VECTOR('',#49036,1000.);
#11310=VECTOR('',#49051,1000.);
#11311=VECTOR('',#49060,1000.);
#11312=VECTOR('',#49077,1000.);
#11313=VECTOR('',#49078,1000.);
#11314=VECTOR('',#49081,1000.);
#11315=VECTOR('',#49082,1000.);
#11316=VECTOR('',#49085,1000.);
#13490=CIRCLE('',#38349,4.64715395326);
#13491=CIRCLE('',#38350,4.64715395326);
#13492=CIRCLE('',#38351,4.64715395326);
#13493=CIRCLE('',#38352,0.3);
#13494=CIRCLE('',#38353,4.35610046976);
#13495=CIRCLE('',#38354,0.3);
#13496=CIRCLE('',#38356,8.85);
#13497=CIRCLE('',#38357,7.28184557105);
#13498=CIRCLE('',#38361,7.28184557105);
#13499=CIRCLE('',#38364,8.85);
#13500=CIRCLE('',#38369,1.2046272227);
#13501=CIRCLE('',#38371,1.2046272227);
#13502=CIRCLE('',#38373,1.8);
#13503=CIRCLE('',#38374,7.35);
#13504=CIRCLE('',#38375,1.8);
#13505=CIRCLE('',#38376,8.85);
#13506=CIRCLE('',#38377,10.8);
#13507=CIRCLE('',#38378,1.8);
#13508=CIRCLE('',#38379,1.8);
#13509=CIRCLE('',#38380,13.5204936174);
#13510=CIRCLE('',#38381,1.8);
#13511=CIRCLE('',#38382,14.05);
#13512=CIRCLE('',#38383,1.8);
#13513=CIRCLE('',#38384,13.5204936174);
#13514=CIRCLE('',#38385,1.8);
#13515=CIRCLE('',#38386,1.8);
#13516=CIRCLE('',#38387,10.8);
#13517=CIRCLE('',#38388,8.85);
#13518=CIRCLE('',#38389,1.8);
#13519=CIRCLE('',#38390,7.35);
#13520=CIRCLE('',#38391,1.8);
#13521=CIRCLE('',#38393,4.19792065612);
#13522=CIRCLE('',#38395,0.3);
#13523=CIRCLE('',#38396,0.3);
#13524=CIRCLE('',#38397,0.3);
#13525=CIRCLE('',#38398,0.3);
#13526=CIRCLE('',#38399,8.85);
#13527=CIRCLE('',#38400,8.85);
#13528=CIRCLE('',#38401,8.85);
#13529=CIRCLE('',#38404,1.5);
#13530=CIRCLE('',#38406,2.54997399005);
#13531=CIRCLE('',#38408,8.85);
#13532=CIRCLE('',#38413,8.85);
#13533=CIRCLE('',#38415,8.85);
#13534=CIRCLE('',#38417,2.55);
#13535=CIRCLE('',#38421,8.85);
#13536=CIRCLE('',#38423,2.55);
#13537=CIRCLE('',#38425,8.85);
#13538=CIRCLE('',#38429,8.85);
#13539=CIRCLE('',#38431,8.85);
#13540=CIRCLE('',#38433,2.54997399005);
#13541=CIRCLE('',#38438,8.85);
#13542=CIRCLE('',#38440,7.35);
#13543=CIRCLE('',#38442,7.35);
#13544=CIRCLE('',#38446,8.85);
#13545=CIRCLE('',#38447,1.8);
#13546=CIRCLE('',#38448,1.8);
#13547=CIRCLE('',#38452,8.85);
#13548=CIRCLE('',#38454,1.8);
#13549=CIRCLE('',#38457,1.8);
#13550=CIRCLE('',#38459,1.5);
#13551=CIRCLE('',#38461,8.85);
#13552=CIRCLE('',#38464,2.54997399005);
#13553=CIRCLE('',#38468,2.54997399005);
#13554=CIRCLE('',#38471,8.85);
#13555=CIRCLE('',#38473,8.85);
#13556=CIRCLE('',#38475,2.55);
#13557=CIRCLE('',#38478,8.85);
#13558=CIRCLE('',#38480,2.55);
#13559=CIRCLE('',#38483,0.3);
#13560=CIRCLE('',#38484,0.3);
#13561=CIRCLE('',#38486,12.3);
#13562=CIRCLE('',#38487,0.3);
#13563=CIRCLE('',#38488,0.3);
#13564=CIRCLE('',#38489,15.55);
#13565=CIRCLE('',#38490,0.3);
#13566=CIRCLE('',#38491,0.3);
#13567=CIRCLE('',#38492,15.0204936174);
#13568=CIRCLE('',#38493,0.3);
#13569=CIRCLE('',#38494,0.3);
#13570=CIRCLE('',#38495,15.55);
#13571=CIRCLE('',#38496,0.3);
#13572=CIRCLE('',#38497,0.3);
#13573=CIRCLE('',#38498,15.0204936174);
#13574=CIRCLE('',#38499,0.3);
#13575=CIRCLE('',#38500,0.3);
#13576=CIRCLE('',#38501,15.55);
#13577=CIRCLE('',#38502,0.3);
#13578=CIRCLE('',#38503,0.3);
#13579=CIRCLE('',#38504,12.3);
#13580=CIRCLE('',#38505,10.35);
#13581=CIRCLE('',#38506,0.6);
#13582=CIRCLE('',#38507,0.6);
#13583=CIRCLE('',#38508,0.6);
#13584=CIRCLE('',#38509,0.6);
#13585=CIRCLE('',#38511,12.3);
#13586=CIRCLE('',#38514,10.35);
#13587=CIRCLE('',#38517,12.3);
#13588=CIRCLE('',#38519,0.3);
#13589=CIRCLE('',#38522,0.3);
#13590=CIRCLE('',#38524,15.55);
#13591=CIRCLE('',#38526,0.3);
#13592=CIRCLE('',#38528,0.3);
#13593=CIRCLE('',#38530,15.0204936174);
#13594=CIRCLE('',#38532,0.3);
#13595=CIRCLE('',#38535,0.3);
#13596=CIRCLE('',#38537,15.55);
#13597=CIRCLE('',#38539,0.3);
#13598=CIRCLE('',#38542,0.3);
#13599=CIRCLE('',#38544,15.0204936174);
#13600=CIRCLE('',#38546,0.3);
#13601=CIRCLE('',#38548,0.3);
#13602=CIRCLE('',#38550,15.55);
#13603=CIRCLE('',#38552,0.3);
#13604=CIRCLE('',#38555,0.3);
#13605=CIRCLE('',#38557,8.85);
#13606=CIRCLE('',#38561,8.85);
#13607=CIRCLE('',#38563,8.85);
#13608=CIRCLE('',#38566,8.85);
#13609=CIRCLE('',#38567,8.85);
#13610=CIRCLE('',#38571,0.3);
#13611=CIRCLE('',#38572,0.300000000000002);
#13612=CIRCLE('',#38575,0.300000000000002);
#13613=CIRCLE('',#38578,0.3);
#13614=CIRCLE('',#38579,0.3);
#13615=CIRCLE('',#38582,0.3);
#13616=CIRCLE('',#38584,0.3);
#13617=CIRCLE('',#38585,0.300092356025301);
#13618=CIRCLE('',#38587,0.3);
#13619=CIRCLE('',#38589,0.3);
#13620=CIRCLE('',#38592,4.47840533247);
#13621=CIRCLE('',#38593,0.300092357885528);
#13622=CIRCLE('',#38595,0.3);
#13623=CIRCLE('',#38597,0.3);
#13624=CIRCLE('',#38599,0.3);
#16432=VERTEX_POINT('',#97332);
#16433=VERTEX_POINT('',#97333);
#16434=VERTEX_POINT('',#97335);
#16435=VERTEX_POINT('',#97337);
#16436=VERTEX_POINT('',#97339);
#16437=VERTEX_POINT('',#97341);
#16438=VERTEX_POINT('',#97345);
#16439=VERTEX_POINT('',#97346);
#16440=VERTEX_POINT('',#97348);
#16441=VERTEX_POINT('',#97350);
#16442=VERTEX_POINT('',#97352);
#16443=VERTEX_POINT('',#97356);
#16444=VERTEX_POINT('',#97358);
#16445=VERTEX_POINT('',#97362);
#16446=VERTEX_POINT('',#97366);
#16447=VERTEX_POINT('',#97370);
#16448=VERTEX_POINT('',#97374);
#16449=VERTEX_POINT('',#97375);
#16450=VERTEX_POINT('',#97377);
#16451=VERTEX_POINT('',#97379);
#16452=VERTEX_POINT('',#97383);
#16453=VERTEX_POINT('',#97384);
#16454=VERTEX_POINT('',#97389);
#16455=VERTEX_POINT('',#97393);
#16456=VERTEX_POINT('',#97397);
#16457=VERTEX_POINT('',#97400);
#16458=VERTEX_POINT('',#97404);
#16459=VERTEX_POINT('',#97406);
#16460=VERTEX_POINT('',#97408);
#16461=VERTEX_POINT('',#97410);
#16462=VERTEX_POINT('',#97412);
#16463=VERTEX_POINT('',#97414);
#16464=VERTEX_POINT('',#97416);
#16465=VERTEX_POINT('',#97418);
#16466=VERTEX_POINT('',#97420);
#16467=VERTEX_POINT('',#97422);
#16468=VERTEX_POINT('',#97424);
#16469=VERTEX_POINT('',#97426);
#16470=VERTEX_POINT('',#97428);
#16471=VERTEX_POINT('',#97430);
#16472=VERTEX_POINT('',#97432);
#16473=VERTEX_POINT('',#97434);
#16474=VERTEX_POINT('',#97436);
#16475=VERTEX_POINT('',#97438);
#16476=VERTEX_POINT('',#97440);
#16477=VERTEX_POINT('',#97442);
#16478=VERTEX_POINT('',#97444);
#16479=VERTEX_POINT('',#97446);
#16480=VERTEX_POINT('',#97448);
#16481=VERTEX_POINT('',#97450);
#16482=VERTEX_POINT('',#97452);
#16483=VERTEX_POINT('',#97454);
#16484=VERTEX_POINT('',#97456);
#16485=VERTEX_POINT('',#97458);
#16486=VERTEX_POINT('',#97462);
#16487=VERTEX_POINT('',#97463);
#16488=VERTEX_POINT('',#97479);
#16489=VERTEX_POINT('',#97481);
#16490=VERTEX_POINT('',#97483);
#16491=VERTEX_POINT('',#97485);
#16492=VERTEX_POINT('',#97487);
#16493=VERTEX_POINT('',#97489);
#16494=VERTEX_POINT('',#97491);
#16495=VERTEX_POINT('',#97493);
#16496=VERTEX_POINT('',#97495);
#16497=VERTEX_POINT('',#97497);
#16498=VERTEX_POINT('',#97499);
#16499=VERTEX_POINT('',#97503);
#16500=VERTEX_POINT('',#97507);
#16501=VERTEX_POINT('',#97508);
#16502=VERTEX_POINT('',#97511);
#16503=VERTEX_POINT('',#97513);
#16504=VERTEX_POINT('',#97518);
#16505=VERTEX_POINT('',#97519);
#16506=VERTEX_POINT('',#97557);
#16507=VERTEX_POINT('',#97561);
#16508=VERTEX_POINT('',#97562);
#16509=VERTEX_POINT('',#97564);
#16510=VERTEX_POINT('',#97566);
#16511=VERTEX_POINT('',#97568);
#16512=VERTEX_POINT('',#97570);
#16513=VERTEX_POINT('',#97574);
#16514=VERTEX_POINT('',#97578);
#16515=VERTEX_POINT('',#97582);
#16516=VERTEX_POINT('',#97595);
#16517=VERTEX_POINT('',#97601);
#16518=VERTEX_POINT('',#97602);
#16519=VERTEX_POINT('',#97604);
#16520=VERTEX_POINT('',#97608);
#16521=VERTEX_POINT('',#97610);
#16522=VERTEX_POINT('',#97612);
#16523=VERTEX_POINT('',#97616);
#16524=VERTEX_POINT('',#97620);
#16525=VERTEX_POINT('',#97635);
#16526=VERTEX_POINT('',#97636);
#16527=VERTEX_POINT('',#97638);
#16528=VERTEX_POINT('',#97640);
#16529=VERTEX_POINT('',#97642);
#16530=VERTEX_POINT('',#97646);
#16531=VERTEX_POINT('',#97650);
#16532=VERTEX_POINT('',#97663);
#16533=VERTEX_POINT('',#97669);
#16534=VERTEX_POINT('',#97670);
#16535=VERTEX_POINT('',#97672);
#16536=VERTEX_POINT('',#97676);
#16537=VERTEX_POINT('',#97678);
#16538=VERTEX_POINT('',#97680);
#16539=VERTEX_POINT('',#97682);
#16540=VERTEX_POINT('',#97686);
#16541=VERTEX_POINT('',#97690);
#16542=VERTEX_POINT('',#97703);
#16543=VERTEX_POINT('',#97709);
#16544=VERTEX_POINT('',#97710);
#16545=VERTEX_POINT('',#97714);
#16546=VERTEX_POINT('',#97715);
#16547=VERTEX_POINT('',#97725);
#16548=VERTEX_POINT('',#97726);
#16549=VERTEX_POINT('',#97728);
#16550=VERTEX_POINT('',#97730);
#16551=VERTEX_POINT('',#97738);
#16552=VERTEX_POINT('',#97739);
#16553=VERTEX_POINT('',#97744);
#16554=VERTEX_POINT('',#97748);
#16555=VERTEX_POINT('',#97754);
#16556=VERTEX_POINT('',#97756);
#16557=VERTEX_POINT('',#97758);
#16558=VERTEX_POINT('',#97797);
#16559=VERTEX_POINT('',#97798);
#16560=VERTEX_POINT('',#97800);
#16561=VERTEX_POINT('',#97804);
#16562=VERTEX_POINT('',#97806);
#16563=VERTEX_POINT('',#97810);
#16564=VERTEX_POINT('',#97821);
#16565=VERTEX_POINT('',#97825);
#16566=VERTEX_POINT('',#97826);
#16567=VERTEX_POINT('',#97831);
#16568=VERTEX_POINT('',#97832);
#16569=VERTEX_POINT('',#97834);
#16570=VERTEX_POINT('',#97836);
#16571=VERTEX_POINT('',#97840);
#16572=VERTEX_POINT('',#97851);
#16573=VERTEX_POINT('',#97855);
#16574=VERTEX_POINT('',#97857);
#16575=VERTEX_POINT('',#97861);
#16576=VERTEX_POINT('',#97865);
#16577=VERTEX_POINT('',#97866);
#16578=VERTEX_POINT('',#97868);
#16579=VERTEX_POINT('',#97872);
#16580=VERTEX_POINT('',#97883);
#16581=VERTEX_POINT('',#97887);
#16582=VERTEX_POINT('',#97889);
#16583=VERTEX_POINT('',#97893);
#16584=VERTEX_POINT('',#97894);
#16585=VERTEX_POINT('',#97896);
#16586=VERTEX_POINT('',#97900);
#16587=VERTEX_POINT('',#97901);
#16588=VERTEX_POINT('',#97915);
#16589=VERTEX_POINT('',#97917);
#16590=VERTEX_POINT('',#97921);
#16591=VERTEX_POINT('',#97923);
#16592=VERTEX_POINT('',#97927);
#16593=VERTEX_POINT('',#97928);
#16594=VERTEX_POINT('',#97930);
#16595=VERTEX_POINT('',#97932);
#16596=VERTEX_POINT('',#97934);
#16597=VERTEX_POINT('',#97936);
#16598=VERTEX_POINT('',#97938);
#16599=VERTEX_POINT('',#97940);
#16600=VERTEX_POINT('',#97942);
#16601=VERTEX_POINT('',#97944);
#16602=VERTEX_POINT('',#97946);
#16603=VERTEX_POINT('',#97948);
#16604=VERTEX_POINT('',#97950);
#16605=VERTEX_POINT('',#97952);
#16606=VERTEX_POINT('',#97954);
#16607=VERTEX_POINT('',#97956);
#16608=VERTEX_POINT('',#97958);
#16609=VERTEX_POINT('',#97960);
#16610=VERTEX_POINT('',#97962);
#16611=VERTEX_POINT('',#97964);
#16612=VERTEX_POINT('',#97966);
#16613=VERTEX_POINT('',#97968);
#16614=VERTEX_POINT('',#97970);
#16615=VERTEX_POINT('',#97972);
#16616=VERTEX_POINT('',#97974);
#16617=VERTEX_POINT('',#97976);
#16618=VERTEX_POINT('',#97980);
#16619=VERTEX_POINT('',#97982);
#16620=VERTEX_POINT('',#97984);
#16621=VERTEX_POINT('',#97986);
#16622=VERTEX_POINT('',#97990);
#16623=VERTEX_POINT('',#97992);
#16624=VERTEX_POINT('',#97996);
#16625=VERTEX_POINT('',#98000);
#16626=VERTEX_POINT('',#98004);
#16627=VERTEX_POINT('',#98008);
#16628=VERTEX_POINT('',#98012);
#16629=VERTEX_POINT('',#98016);
#16630=VERTEX_POINT('',#98020);
#16631=VERTEX_POINT('',#98024);
#16632=VERTEX_POINT('',#98028);
#16633=VERTEX_POINT('',#98032);
#16634=VERTEX_POINT('',#98036);
#16635=VERTEX_POINT('',#98040);
#16636=VERTEX_POINT('',#98044);
#16637=VERTEX_POINT('',#98048);
#16638=VERTEX_POINT('',#98052);
#16639=VERTEX_POINT('',#98056);
#16640=VERTEX_POINT('',#98060);
#16641=VERTEX_POINT('',#98064);
#16642=VERTEX_POINT('',#98068);
#16643=VERTEX_POINT('',#98072);
#16644=VERTEX_POINT('',#98076);
#16645=VERTEX_POINT('',#98080);
#16646=VERTEX_POINT('',#98084);
#16647=VERTEX_POINT('',#98088);
#16648=VERTEX_POINT('',#98094);
#16649=VERTEX_POINT('',#98100);
#16650=VERTEX_POINT('',#98106);
#16651=VERTEX_POINT('',#98112);
#16652=VERTEX_POINT('',#98115);
#16653=VERTEX_POINT('',#98122);
#16654=VERTEX_POINT('',#98128);
#16655=VERTEX_POINT('',#98134);
#16656=VERTEX_POINT('',#98140);
#16657=VERTEX_POINT('',#98181);
#16658=VERTEX_POINT('',#98183);
#16659=VERTEX_POINT('',#98202);
#16660=VERTEX_POINT('',#98243);
#16661=VERTEX_POINT('',#98259);
#16662=VERTEX_POINT('',#98263);
#21439=EDGE_CURVE('',#16432,#16433,#13490,.T.);
#21440=EDGE_CURVE('',#16433,#16434,#13491,.T.);
#21441=EDGE_CURVE('',#16434,#16435,#13492,.T.);
#21442=EDGE_CURVE('',#16436,#16435,#13493,.T.);
#21443=EDGE_CURVE('',#16437,#16436,#13494,.T.);
#21444=EDGE_CURVE('',#16437,#16432,#13495,.T.);
#21445=EDGE_CURVE('',#16438,#16439,#13496,.T.);
#21446=EDGE_CURVE('',#16439,#16440,#9284,.T.);
#21447=EDGE_CURVE('',#16440,#16441,#13497,.T.);
#21448=EDGE_CURVE('',#16441,#16442,#9285,.T.);
#21449=EDGE_CURVE('',#16442,#16438,#9286,.T.);
#21450=EDGE_CURVE('',#16443,#16442,#9287,.T.);
#21451=EDGE_CURVE('',#16443,#16444,#9288,.T.);
#21452=EDGE_CURVE('',#16444,#16438,#9289,.T.);
#21453=EDGE_CURVE('',#16445,#16441,#9290,.T.);
#21454=EDGE_CURVE('',#16445,#16443,#9291,.T.);
#21455=EDGE_CURVE('',#16446,#16440,#9292,.T.);
#21456=EDGE_CURVE('',#16446,#16445,#13498,.T.);
#21457=EDGE_CURVE('',#16447,#16439,#9293,.T.);
#21458=EDGE_CURVE('',#16447,#16446,#9294,.T.);
#21459=EDGE_CURVE('',#16448,#16449,#9295,.T.);
#21460=EDGE_CURVE('',#16450,#16448,#9296,.T.);
#21461=EDGE_CURVE('',#16450,#16451,#13499,.T.);
#21462=EDGE_CURVE('',#16449,#16451,#9297,.T.);
#21463=EDGE_CURVE('',#16452,#16453,#9298,.T.);
#21464=EDGE_CURVE('',#16453,#16450,#9299,.T.);
#21465=EDGE_CURVE('',#16452,#16448,#9300,.T.);
#21466=EDGE_CURVE('',#16454,#16449,#9301,.T.);
#21467=EDGE_CURVE('',#16454,#16452,#9302,.T.);
#21468=EDGE_CURVE('',#16455,#16451,#9303,.T.);
#21469=EDGE_CURVE('',#16455,#16454,#9304,.T.);
#21470=EDGE_CURVE('',#16456,#16456,#13500,.T.);
#21471=EDGE_CURVE('',#16456,#16457,#9305,.T.);
#21472=EDGE_CURVE('',#16457,#16457,#13501,.T.);
#21473=EDGE_CURVE('',#16433,#16458,#9306,.T.);
#21474=EDGE_CURVE('',#16459,#16458,#13502,.T.);
#21475=EDGE_CURVE('',#16460,#16459,#9307,.T.);
#21476=EDGE_CURVE('',#16460,#16461,#13503,.T.);
#21477=EDGE_CURVE('',#16462,#16461,#9308,.T.);
#21478=EDGE_CURVE('',#16463,#16462,#13504,.T.);
#21479=EDGE_CURVE('',#16464,#16463,#13505,.T.);
#21480=EDGE_CURVE('',#16464,#16465,#9309,.T.);
#21481=EDGE_CURVE('',#16465,#16466,#13506,.T.);
#21482=EDGE_CURVE('',#16467,#16466,#13507,.T.);
#21483=EDGE_CURVE('',#16467,#16468,#9310,.T.);
#21484=EDGE_CURVE('',#16468,#16469,#13508,.T.);
#21485=EDGE_CURVE('',#16470,#16469,#13509,.T.);
#21486=EDGE_CURVE('',#16471,#16470,#13510,.T.);
#21487=EDGE_CURVE('',#16471,#16472,#13511,.T.);
#21488=EDGE_CURVE('',#16472,#16473,#13512,.T.);
#21489=EDGE_CURVE('',#16474,#16473,#13513,.T.);
#21490=EDGE_CURVE('',#16474,#16475,#13514,.T.);
#21491=EDGE_CURVE('',#16476,#16475,#9311,.T.);
#21492=EDGE_CURVE('',#16476,#16477,#13515,.T.);
#21493=EDGE_CURVE('',#16477,#16478,#13516,.T.);
#21494=EDGE_CURVE('',#16478,#16479,#9312,.T.);
#21495=EDGE_CURVE('',#16480,#16479,#13517,.T.);
#21496=EDGE_CURVE('',#16481,#16480,#13518,.T.);
#21497=EDGE_CURVE('',#16481,#16482,#9313,.T.);
#21498=EDGE_CURVE('',#16482,#16483,#13519,.T.);
#21499=EDGE_CURVE('',#16483,#16484,#9314,.T.);
#21500=EDGE_CURVE('',#16485,#16484,#13520,.T.);
#21501=EDGE_CURVE('',#16485,#16434,#9315,.T.);
#21502=EDGE_CURVE('',#16486,#16487,#13521,.T.);
#21503=EDGE_CURVE('',#16487,#16437,#2027,.T.);
#21504=EDGE_CURVE('',#16436,#16486,#2028,.T.);
#21505=EDGE_CURVE('',#16488,#16445,#13522,.T.);
#21506=EDGE_CURVE('',#16488,#16489,#9316,.T.);
#21507=EDGE_CURVE('',#16490,#16489,#13523,.T.);
#21508=EDGE_CURVE('',#16490,#16491,#9317,.T.);
#21509=EDGE_CURVE('',#16491,#16492,#9318,.T.);
#21510=EDGE_CURVE('',#16492,#16493,#9319,.T.);
#21511=EDGE_CURVE('',#16494,#16493,#9320,.T.);
#21512=EDGE_CURVE('',#16494,#16495,#9321,.T.);
#21513=EDGE_CURVE('',#16496,#16495,#13524,.T.);
#21514=EDGE_CURVE('',#16497,#16496,#9322,.T.);
#21515=EDGE_CURVE('',#16498,#16497,#13525,.T.);
#21516=EDGE_CURVE('',#16445,#16498,#9323,.T.);
#21517=EDGE_CURVE('',#16447,#16453,#13526,.T.);
#21518=EDGE_CURVE('',#16455,#16499,#13527,.T.);
#21519=EDGE_CURVE('',#16499,#16444,#13528,.T.);
#21520=EDGE_CURVE('',#16500,#16501,#9324,.T.);
#21521=EDGE_CURVE('',#16495,#16500,#9325,.T.);
#21522=EDGE_CURVE('',#16494,#16502,#9326,.T.);
#21523=EDGE_CURVE('',#16503,#16502,#9327,.T.);
#21524=EDGE_CURVE('',#16491,#16503,#9328,.T.);
#21525=EDGE_CURVE('',#16490,#16501,#9329,.T.);
#21526=EDGE_CURVE('',#16504,#16505,#2029,.T.);
#21527=EDGE_CURVE('',#16505,#16504,#2030,.T.);
#21528=EDGE_CURVE('',#16505,#16506,#9330,.T.);
#21529=EDGE_CURVE('',#16506,#16506,#13529,.T.);
#21530=EDGE_CURVE('',#16507,#16508,#9331,.T.);
#21531=EDGE_CURVE('',#16507,#16509,#9332,.T.);
#21532=EDGE_CURVE('',#16509,#16510,#9333,.T.);
#21533=EDGE_CURVE('',#16510,#16511,#13530,.T.);
#21534=EDGE_CURVE('',#16512,#16511,#9334,.T.);
#21535=EDGE_CURVE('',#16512,#16508,#9335,.T.);
#21536=EDGE_CURVE('',#16512,#16513,#9336,.T.);
#21537=EDGE_CURVE('',#16508,#16513,#13531,.T.);
#21538=EDGE_CURVE('',#16513,#16514,#9337,.T.);
#21539=EDGE_CURVE('',#16514,#16511,#9338,.T.);
#21540=EDGE_CURVE('',#16515,#16514,#2031,.T.);
#21541=EDGE_CURVE('',#16510,#16515,#9339,.T.);
#21542=EDGE_CURVE('',#16515,#16516,#9340,.T.);
#21543=EDGE_CURVE('',#16509,#16516,#9341,.T.);
#21544=EDGE_CURVE('',#16507,#16516,#13532,.T.);
#21545=EDGE_CURVE('',#16517,#16518,#13533,.T.);
#21546=EDGE_CURVE('',#16518,#16519,#9342,.T.);
#21547=EDGE_CURVE('',#16519,#16517,#9343,.T.);
#21548=EDGE_CURVE('',#16520,#16518,#9344,.T.);
#21549=EDGE_CURVE('',#16521,#16520,#9345,.T.);
#21550=EDGE_CURVE('',#16521,#16522,#13534,.T.);
#21551=EDGE_CURVE('',#16522,#16519,#9346,.T.);
#21552=EDGE_CURVE('',#16517,#16523,#9347,.T.);
#21553=EDGE_CURVE('',#16523,#16522,#9348,.T.);
#21554=EDGE_CURVE('',#16521,#16524,#9349,.T.);
#21555=EDGE_CURVE('',#16524,#16523,#2032,.T.);
#21556=EDGE_CURVE('',#16520,#16524,#13535,.T.);
#21557=EDGE_CURVE('',#16525,#16526,#9350,.T.);
#21558=EDGE_CURVE('',#16527,#16526,#9351,.T.);
#21559=EDGE_CURVE('',#16528,#16527,#9352,.T.);
#21560=EDGE_CURVE('',#16528,#16529,#13536,.T.);
#21561=EDGE_CURVE('',#16525,#16529,#9353,.T.);
#21562=EDGE_CURVE('',#16530,#16525,#13537,.T.);
#21563=EDGE_CURVE('',#16529,#16530,#9354,.T.);
#21564=EDGE_CURVE('',#16531,#16528,#9355,.T.);
#21565=EDGE_CURVE('',#16530,#16531,#2033,.T.);
#21566=EDGE_CURVE('',#16527,#16532,#9356,.T.);
#21567=EDGE_CURVE('',#16532,#16531,#9357,.T.);
#21568=EDGE_CURVE('',#16526,#16532,#13538,.T.);
#21569=EDGE_CURVE('',#16533,#16534,#13539,.T.);
#21570=EDGE_CURVE('',#16535,#16534,#9358,.T.);
#21571=EDGE_CURVE('',#16535,#16533,#9359,.T.);
#21572=EDGE_CURVE('',#16534,#16536,#9360,.T.);
#21573=EDGE_CURVE('',#16536,#16537,#9361,.T.);
#21574=EDGE_CURVE('',#16537,#16538,#9362,.T.);
#21575=EDGE_CURVE('',#16538,#16539,#13540,.T.);
#21576=EDGE_CURVE('',#16535,#16539,#9363,.T.);
#21577=EDGE_CURVE('',#16539,#16540,#9364,.T.);
#21578=EDGE_CURVE('',#16540,#16533,#9365,.T.);
#21579=EDGE_CURVE('',#16541,#16540,#2034,.T.);
#21580=EDGE_CURVE('',#16541,#16538,#9366,.T.);
#21581=EDGE_CURVE('',#16542,#16541,#9367,.T.);
#21582=EDGE_CURVE('',#16537,#16542,#9368,.T.);
#21583=EDGE_CURVE('',#16542,#16536,#13541,.T.);
#21584=EDGE_CURVE('',#16543,#16544,#13542,.T.);
#21585=EDGE_CURVE('',#16543,#16544,#9369,.T.);
#21586=EDGE_CURVE('',#16545,#16546,#13543,.T.);
#21587=EDGE_CURVE('',#16546,#16545,#9370,.T.);
#21588=EDGE_CURVE('',#16546,#16482,#9371,.T.);
#21589=EDGE_CURVE('',#16483,#16545,#9372,.T.);
#21590=EDGE_CURVE('',#16543,#16461,#9373,.T.);
#21591=EDGE_CURVE('',#16460,#16544,#9374,.T.);
#21592=EDGE_CURVE('',#16547,#16548,#13544,.T.);
#21593=EDGE_CURVE('',#16549,#16547,#13545,.T.);
#21594=EDGE_CURVE('',#16550,#16549,#9375,.T.);
#21595=EDGE_CURVE('',#16548,#16550,#13546,.T.);
#21596=EDGE_CURVE('',#16461,#16460,#9376,.T.);
#21597=EDGE_CURVE('',#16482,#16483,#9377,.T.);
#21598=EDGE_CURVE('',#16551,#16552,#13547,.T.);
#21599=EDGE_CURVE('',#16551,#16547,#9378,.T.);
#21600=EDGE_CURVE('',#16548,#16552,#9379,.T.);
#21601=EDGE_CURVE('',#16552,#16553,#13548,.T.);
#21602=EDGE_CURVE('',#16550,#16553,#9380,.T.);
#21603=EDGE_CURVE('',#16549,#16554,#9381,.T.);
#21604=EDGE_CURVE('',#16553,#16554,#9382,.T.);
#21605=EDGE_CURVE('',#16554,#16551,#13549,.T.);
#21606=EDGE_CURVE('',#16555,#16555,#13550,.T.);
#21607=EDGE_CURVE('',#16555,#16556,#9383,.T.);
#21608=EDGE_CURVE('',#16556,#16557,#2035,.T.);
#21609=EDGE_CURVE('',#16557,#16556,#2036,.T.);
#21610=EDGE_CURVE('',#16558,#16559,#13551,.T.);
#21611=EDGE_CURVE('',#16560,#16559,#9384,.T.);
#21612=EDGE_CURVE('',#16560,#16558,#9385,.T.);
#21613=EDGE_CURVE('',#16559,#16561,#9386,.T.);
#21614=EDGE_CURVE('',#16561,#16562,#9387,.T.);
#21615=EDGE_CURVE('',#16560,#16562,#9388,.T.);
#21616=EDGE_CURVE('',#16563,#16561,#2037,.T.);
#21617=EDGE_CURVE('',#16564,#16563,#9389,.T.);
#21618=EDGE_CURVE('',#16564,#16562,#13552,.T.);
#21619=EDGE_CURVE('',#16565,#16566,#9390,.T.);
#21620=EDGE_CURVE('',#16566,#16564,#9391,.T.);
#21621=EDGE_CURVE('',#16563,#16565,#9392,.T.);
#21622=EDGE_CURVE('',#16567,#16568,#9393,.T.);
#21623=EDGE_CURVE('',#16569,#16567,#9394,.T.);
#21624=EDGE_CURVE('',#16570,#16569,#9395,.T.);
#21625=EDGE_CURVE('',#16568,#16570,#9396,.T.);
#21626=EDGE_CURVE('',#16571,#16567,#2038,.T.);
#21627=EDGE_CURVE('',#16571,#16572,#9397,.T.);
#21628=EDGE_CURVE('',#16572,#16569,#13553,.T.);
#21629=EDGE_CURVE('',#16573,#16572,#9398,.T.);
#21630=EDGE_CURVE('',#16574,#16571,#9399,.T.);
#21631=EDGE_CURVE('',#16573,#16574,#9400,.T.);
#21632=EDGE_CURVE('',#16574,#16575,#13554,.T.);
#21633=EDGE_CURVE('',#16575,#16573,#9401,.T.);
#21634=EDGE_CURVE('',#16576,#16577,#9402,.T.);
#21635=EDGE_CURVE('',#16578,#16576,#13555,.T.);
#21636=EDGE_CURVE('',#16577,#16578,#9403,.T.);
#21637=EDGE_CURVE('',#16578,#16579,#2039,.T.);
#21638=EDGE_CURVE('',#16579,#16580,#9404,.T.);
#21639=EDGE_CURVE('',#16580,#16577,#13556,.T.);
#21640=EDGE_CURVE('',#16581,#16579,#9405,.T.);
#21641=EDGE_CURVE('',#16581,#16582,#9406,.T.);
#21642=EDGE_CURVE('',#16580,#16582,#9407,.T.);
#21643=EDGE_CURVE('',#16583,#16584,#9408,.T.);
#21644=EDGE_CURVE('',#16583,#16585,#9409,.T.);
#21645=EDGE_CURVE('',#16584,#16585,#13557,.T.);
#21646=EDGE_CURVE('',#16586,#16587,#9410,.T.);
#21647=EDGE_CURVE('',#16585,#16586,#2040,.T.);
#21648=EDGE_CURVE('',#16583,#16587,#13558,.T.);
#21649=EDGE_CURVE('',#16587,#16588,#9411,.T.);
#21650=EDGE_CURVE('',#16589,#16588,#9412,.T.);
#21651=EDGE_CURVE('',#16589,#16586,#9413,.T.);
#21652=EDGE_CURVE('',#16590,#16500,#13559,.T.);
#21653=EDGE_CURVE('',#16591,#16501,#13560,.T.);
#21654=EDGE_CURVE('',#16590,#16591,#9414,.T.);
#21655=EDGE_CURVE('',#16592,#16593,#9415,.T.);
#21656=EDGE_CURVE('',#16593,#16594,#13561,.T.);
#21657=EDGE_CURVE('',#16594,#16595,#13562,.T.);
#21658=EDGE_CURVE('',#16595,#16596,#9416,.T.);
#21659=EDGE_CURVE('',#16597,#16596,#13563,.T.);
#21660=EDGE_CURVE('',#16597,#16598,#13564,.T.);
#21661=EDGE_CURVE('',#16599,#16598,#13565,.T.);
#21662=EDGE_CURVE('',#16599,#16600,#13566,.T.);
#21663=EDGE_CURVE('',#16600,#16601,#13567,.T.);
#21664=EDGE_CURVE('',#16601,#16602,#13568,.T.);
#21665=EDGE_CURVE('',#16602,#16603,#9417,.T.);
#21666=EDGE_CURVE('',#16604,#16603,#13569,.T.);
#21667=EDGE_CURVE('',#16604,#16605,#13570,.T.);
#21668=EDGE_CURVE('',#16606,#16605,#13571,.T.);
#21669=EDGE_CURVE('',#16606,#16607,#9418,.T.);
#21670=EDGE_CURVE('',#16607,#16608,#13572,.T.);
#21671=EDGE_CURVE('',#16608,#16609,#13573,.T.);
#21672=EDGE_CURVE('',#16609,#16610,#13574,.T.);
#21673=EDGE_CURVE('',#16611,#16610,#13575,.T.);
#21674=EDGE_CURVE('',#16611,#16612,#13576,.T.);
#21675=EDGE_CURVE('',#16613,#16612,#13577,.T.);
#21676=EDGE_CURVE('',#16614,#16613,#9419,.T.);
#21677=EDGE_CURVE('',#16614,#16615,#13578,.T.);
#21678=EDGE_CURVE('',#16615,#16616,#13579,.T.);
#21679=EDGE_CURVE('',#16616,#16617,#9420,.T.);
#21680=EDGE_CURVE('',#16617,#16592,#13580,.T.);
#21681=EDGE_CURVE('',#16432,#16590,#13581,.T.);
#21682=EDGE_CURVE('',#16591,#16618,#13582,.T.);
#21683=EDGE_CURVE('',#16618,#16619,#9421,.T.);
#21684=EDGE_CURVE('',#16619,#16620,#13583,.T.);
#21685=EDGE_CURVE('',#16620,#16621,#9422,.T.);
#21686=EDGE_CURVE('',#16621,#16435,#13584,.T.);
#21687=EDGE_CURVE('',#16622,#16594,#9423,.T.);
#21688=EDGE_CURVE('',#16593,#16623,#9424,.T.);
#21689=EDGE_CURVE('',#16623,#16622,#13585,.T.);
#21690=EDGE_CURVE('',#16624,#16592,#9425,.T.);
#21691=EDGE_CURVE('',#16624,#16623,#9426,.T.);
#21692=EDGE_CURVE('',#16625,#16624,#13586,.T.);
#21693=EDGE_CURVE('',#16625,#16617,#9427,.T.);
#21694=EDGE_CURVE('',#16616,#16626,#9428,.T.);
#21695=EDGE_CURVE('',#16626,#16625,#9429,.T.);
#21696=EDGE_CURVE('',#16627,#16615,#9430,.T.);
#21697=EDGE_CURVE('',#16627,#16626,#13587,.T.);
#21698=EDGE_CURVE('',#16628,#16614,#9431,.T.);
#21699=EDGE_CURVE('',#16627,#16628,#13588,.T.);
#21700=EDGE_CURVE('',#16613,#16629,#9432,.T.);
#21701=EDGE_CURVE('',#16629,#16628,#9433,.T.);
#21702=EDGE_CURVE('',#16630,#16629,#13589,.T.);
#21703=EDGE_CURVE('',#16612,#16630,#9434,.T.);
#21704=EDGE_CURVE('',#16631,#16630,#13590,.T.);
#21705=EDGE_CURVE('',#16611,#16631,#9435,.T.);
#21706=EDGE_CURVE('',#16632,#16631,#13591,.T.);
#21707=EDGE_CURVE('',#16632,#16610,#9436,.T.);
#21708=EDGE_CURVE('',#16633,#16609,#9437,.T.);
#21709=EDGE_CURVE('',#16632,#16633,#13592,.T.);
#21710=EDGE_CURVE('',#16634,#16608,#9438,.T.);
#21711=EDGE_CURVE('',#16634,#16633,#13593,.T.);
#21712=EDGE_CURVE('',#16635,#16607,#9439,.T.);
#21713=EDGE_CURVE('',#16634,#16635,#13594,.T.);
#21714=EDGE_CURVE('',#16636,#16635,#9440,.T.);
#21715=EDGE_CURVE('',#16606,#16636,#9441,.T.);
#21716=EDGE_CURVE('',#16637,#16636,#13595,.T.);
#21717=EDGE_CURVE('',#16605,#16637,#9442,.T.);
#21718=EDGE_CURVE('',#16604,#16638,#9443,.T.);
#21719=EDGE_CURVE('',#16638,#16637,#13596,.T.);
#21720=EDGE_CURVE('',#16639,#16638,#13597,.T.);
#21721=EDGE_CURVE('',#16603,#16639,#9444,.T.);
#21722=EDGE_CURVE('',#16640,#16602,#9445,.T.);
#21723=EDGE_CURVE('',#16640,#16639,#9446,.T.);
#21724=EDGE_CURVE('',#16641,#16601,#9447,.T.);
#21725=EDGE_CURVE('',#16640,#16641,#13598,.T.);
#21726=EDGE_CURVE('',#16642,#16600,#9448,.T.);
#21727=EDGE_CURVE('',#16642,#16641,#13599,.T.);
#21728=EDGE_CURVE('',#16599,#16643,#9449,.T.);
#21729=EDGE_CURVE('',#16642,#16643,#13600,.T.);
#21730=EDGE_CURVE('',#16644,#16643,#13601,.T.);
#21731=EDGE_CURVE('',#16598,#16644,#9450,.T.);
#21732=EDGE_CURVE('',#16597,#16645,#9451,.T.);
#21733=EDGE_CURVE('',#16645,#16644,#13602,.T.);
#21734=EDGE_CURVE('',#16646,#16645,#13603,.T.);
#21735=EDGE_CURVE('',#16596,#16646,#9452,.T.);
#21736=EDGE_CURVE('',#16647,#16595,#9453,.T.);
#21737=EDGE_CURVE('',#16647,#16646,#9454,.T.);
#21738=EDGE_CURVE('',#16647,#16622,#13604,.T.);
#21739=EDGE_CURVE('',#16581,#16648,#13605,.T.);
#21740=EDGE_CURVE('',#16582,#16648,#9455,.T.);
#21741=EDGE_CURVE('',#16576,#16648,#9456,.T.);
#21742=EDGE_CURVE('',#16649,#16575,#9457,.T.);
#21743=EDGE_CURVE('',#16570,#16649,#9458,.T.);
#21744=EDGE_CURVE('',#16649,#16568,#13606,.T.);
#21745=EDGE_CURVE('',#16565,#16650,#13607,.T.);
#21746=EDGE_CURVE('',#16650,#16566,#9459,.T.);
#21747=EDGE_CURVE('',#16650,#16558,#9460,.T.);
#21748=EDGE_CURVE('',#16499,#16651,#9461,.T.);
#21749=EDGE_CURVE('',#16651,#16651,#13608,.T.);
#21750=EDGE_CURVE('',#16652,#16589,#13609,.T.);
#21751=EDGE_CURVE('',#16584,#16652,#9462,.T.);
#21752=EDGE_CURVE('',#16652,#16588,#9463,.T.);
#21753=EDGE_CURVE('',#16501,#16653,#13610,.T.);
#21754=EDGE_CURVE('',#16618,#16653,#13611,.T.);
#21755=EDGE_CURVE('',#16489,#16653,#9464,.T.);
#21756=EDGE_CURVE('',#16653,#16654,#9465,.T.);
#21757=EDGE_CURVE('',#16619,#16654,#13612,.T.);
#21758=EDGE_CURVE('',#16488,#16654,#9466,.T.);
#21759=EDGE_CURVE('',#16654,#16655,#13613,.T.);
#21760=EDGE_CURVE('',#16620,#16655,#13614,.T.);
#21761=EDGE_CURVE('',#16445,#16655,#9467,.T.);
#21762=EDGE_CURVE('',#16655,#16656,#9468,.T.);
#21763=EDGE_CURVE('',#16621,#16656,#13615,.T.);
#21764=EDGE_CURVE('',#16498,#16656,#9469,.T.);
#21765=EDGE_CURVE('',#16436,#16657,#13616,.T.);
#21766=EDGE_CURVE('',#16657,#16658,#2041,.T.);
#21767=EDGE_CURVE('',#16486,#16658,#13617,.T.);
#21768=EDGE_CURVE('',#16435,#16657,#13618,.T.);
#21769=EDGE_CURVE('',#16656,#16657,#13619,.T.);
#21770=EDGE_CURVE('',#16497,#16658,#9470,.T.);
#21771=EDGE_CURVE('',#16658,#16659,#13620,.T.);
#21772=EDGE_CURVE('',#16487,#16659,#13621,.T.);
#21773=EDGE_CURVE('',#16496,#16659,#9471,.T.);
#21774=EDGE_CURVE('',#16659,#16660,#2042,.T.);
#21775=EDGE_CURVE('',#16437,#16660,#13622,.T.);
#21776=EDGE_CURVE('',#16660,#16432,#13623,.T.);
#21777=EDGE_CURVE('',#16660,#16500,#13624,.T.);
#21778=EDGE_CURVE('',#16661,#16503,#9472,.T.);
#21779=EDGE_CURVE('',#16492,#16661,#9473,.T.);
#21780=EDGE_CURVE('',#16661,#16662,#9474,.T.);
#21781=EDGE_CURVE('',#16493,#16662,#9475,.T.);
#21782=EDGE_CURVE('',#16662,#16502,#9476,.T.);
#31335=ORIENTED_EDGE('',*,*,#21439,.T.);
#31336=ORIENTED_EDGE('',*,*,#21440,.T.);
#31337=ORIENTED_EDGE('',*,*,#21441,.T.);
#31338=ORIENTED_EDGE('',*,*,#21442,.F.);
#31339=ORIENTED_EDGE('',*,*,#21443,.F.);
#31340=ORIENTED_EDGE('',*,*,#21444,.T.);
#31341=ORIENTED_EDGE('',*,*,#21445,.T.);
#31342=ORIENTED_EDGE('',*,*,#21446,.T.);
#31343=ORIENTED_EDGE('',*,*,#21447,.T.);
#31344=ORIENTED_EDGE('',*,*,#21448,.T.);
#31345=ORIENTED_EDGE('',*,*,#21449,.T.);
#31346=ORIENTED_EDGE('',*,*,#21450,.F.);
#31347=ORIENTED_EDGE('',*,*,#21451,.T.);
#31348=ORIENTED_EDGE('',*,*,#21452,.T.);
#31349=ORIENTED_EDGE('',*,*,#21449,.F.);
#31350=ORIENTED_EDGE('',*,*,#21453,.F.);
#31351=ORIENTED_EDGE('',*,*,#21454,.T.);
#31352=ORIENTED_EDGE('',*,*,#21450,.T.);
#31353=ORIENTED_EDGE('',*,*,#21448,.F.);
#31354=ORIENTED_EDGE('',*,*,#21455,.F.);
#31355=ORIENTED_EDGE('',*,*,#21456,.T.);
#31356=ORIENTED_EDGE('',*,*,#21453,.T.);
#31357=ORIENTED_EDGE('',*,*,#21447,.F.);
#31358=ORIENTED_EDGE('',*,*,#21457,.F.);
#31359=ORIENTED_EDGE('',*,*,#21458,.T.);
#31360=ORIENTED_EDGE('',*,*,#21455,.T.);
#31361=ORIENTED_EDGE('',*,*,#21446,.F.);
#31362=ORIENTED_EDGE('',*,*,#21459,.F.);
#31363=ORIENTED_EDGE('',*,*,#21460,.F.);
#31364=ORIENTED_EDGE('',*,*,#21461,.T.);
#31365=ORIENTED_EDGE('',*,*,#21462,.F.);
#31366=ORIENTED_EDGE('',*,*,#21463,.T.);
#31367=ORIENTED_EDGE('',*,*,#21464,.T.);
#31368=ORIENTED_EDGE('',*,*,#21460,.T.);
#31369=ORIENTED_EDGE('',*,*,#21465,.F.);
#31370=ORIENTED_EDGE('',*,*,#21459,.T.);
#31371=ORIENTED_EDGE('',*,*,#21466,.F.);
#31372=ORIENTED_EDGE('',*,*,#21467,.T.);
#31373=ORIENTED_EDGE('',*,*,#21465,.T.);
#31374=ORIENTED_EDGE('',*,*,#21462,.T.);
#31375=ORIENTED_EDGE('',*,*,#21468,.F.);
#31376=ORIENTED_EDGE('',*,*,#21469,.T.);
#31377=ORIENTED_EDGE('',*,*,#21466,.T.);
#31378=ORIENTED_EDGE('',*,*,#21470,.T.);
#31379=ORIENTED_EDGE('',*,*,#21470,.F.);
#31380=ORIENTED_EDGE('',*,*,#21471,.T.);
#31381=ORIENTED_EDGE('',*,*,#21472,.T.);
#31382=ORIENTED_EDGE('',*,*,#21471,.F.);
#31383=ORIENTED_EDGE('',*,*,#21473,.T.);
#31384=ORIENTED_EDGE('',*,*,#21474,.F.);
#31385=ORIENTED_EDGE('',*,*,#21475,.F.);
#31386=ORIENTED_EDGE('',*,*,#21476,.T.);
#31387=ORIENTED_EDGE('',*,*,#21477,.F.);
#31388=ORIENTED_EDGE('',*,*,#21478,.F.);
#31389=ORIENTED_EDGE('',*,*,#21479,.F.);
#31390=ORIENTED_EDGE('',*,*,#21480,.T.);
#31391=ORIENTED_EDGE('',*,*,#21481,.T.);
#31392=ORIENTED_EDGE('',*,*,#21482,.F.);
#31393=ORIENTED_EDGE('',*,*,#21483,.T.);
#31394=ORIENTED_EDGE('',*,*,#21484,.T.);
#31395=ORIENTED_EDGE('',*,*,#21485,.F.);
#31396=ORIENTED_EDGE('',*,*,#21486,.F.);
#31397=ORIENTED_EDGE('',*,*,#21487,.T.);
#31398=ORIENTED_EDGE('',*,*,#21488,.T.);
#31399=ORIENTED_EDGE('',*,*,#21489,.F.);
#31400=ORIENTED_EDGE('',*,*,#21490,.T.);
#31401=ORIENTED_EDGE('',*,*,#21491,.F.);
#31402=ORIENTED_EDGE('',*,*,#21492,.T.);
#31403=ORIENTED_EDGE('',*,*,#21493,.T.);
#31404=ORIENTED_EDGE('',*,*,#21494,.T.);
#31405=ORIENTED_EDGE('',*,*,#21495,.F.);
#31406=ORIENTED_EDGE('',*,*,#21496,.F.);
#31407=ORIENTED_EDGE('',*,*,#21497,.T.);
#31408=ORIENTED_EDGE('',*,*,#21498,.T.);
#31409=ORIENTED_EDGE('',*,*,#21499,.T.);
#31410=ORIENTED_EDGE('',*,*,#21500,.F.);
#31411=ORIENTED_EDGE('',*,*,#21501,.T.);
#31412=ORIENTED_EDGE('',*,*,#21440,.F.);
#31413=ORIENTED_EDGE('',*,*,#21472,.F.);
#31414=ORIENTED_EDGE('',*,*,#21502,.T.);
#31415=ORIENTED_EDGE('',*,*,#21503,.T.);
#31416=ORIENTED_EDGE('',*,*,#21443,.T.);
#31417=ORIENTED_EDGE('',*,*,#21504,.T.);
#31418=ORIENTED_EDGE('',*,*,#21505,.F.);
#31419=ORIENTED_EDGE('',*,*,#21506,.T.);
#31420=ORIENTED_EDGE('',*,*,#21507,.F.);
#31421=ORIENTED_EDGE('',*,*,#21508,.T.);
#31422=ORIENTED_EDGE('',*,*,#21509,.T.);
#31423=ORIENTED_EDGE('',*,*,#21510,.T.);
#31424=ORIENTED_EDGE('',*,*,#21511,.F.);
#31425=ORIENTED_EDGE('',*,*,#21512,.T.);
#31426=ORIENTED_EDGE('',*,*,#21513,.F.);
#31427=ORIENTED_EDGE('',*,*,#21514,.F.);
#31428=ORIENTED_EDGE('',*,*,#21515,.F.);
#31429=ORIENTED_EDGE('',*,*,#21516,.F.);
#31430=ORIENTED_EDGE('',*,*,#21456,.F.);
#31431=ORIENTED_EDGE('',*,*,#21458,.F.);
#31432=ORIENTED_EDGE('',*,*,#21517,.T.);
#31433=ORIENTED_EDGE('',*,*,#21463,.F.);
#31434=ORIENTED_EDGE('',*,*,#21467,.F.);
#31435=ORIENTED_EDGE('',*,*,#21469,.F.);
#31436=ORIENTED_EDGE('',*,*,#21518,.T.);
#31437=ORIENTED_EDGE('',*,*,#21519,.T.);
#31438=ORIENTED_EDGE('',*,*,#21451,.F.);
#31439=ORIENTED_EDGE('',*,*,#21454,.F.);
#31440=ORIENTED_EDGE('',*,*,#21520,.F.);
#31441=ORIENTED_EDGE('',*,*,#21521,.F.);
#31442=ORIENTED_EDGE('',*,*,#21512,.F.);
#31443=ORIENTED_EDGE('',*,*,#21522,.T.);
#31444=ORIENTED_EDGE('',*,*,#21523,.F.);
#31445=ORIENTED_EDGE('',*,*,#21524,.F.);
#31446=ORIENTED_EDGE('',*,*,#21508,.F.);
#31447=ORIENTED_EDGE('',*,*,#21525,.T.);
#31448=ORIENTED_EDGE('',*,*,#21526,.F.);
#31449=ORIENTED_EDGE('',*,*,#21527,.F.);
#31450=ORIENTED_EDGE('',*,*,#21528,.T.);
#31451=ORIENTED_EDGE('',*,*,#21529,.T.);
#31452=ORIENTED_EDGE('',*,*,#21528,.F.);
#31453=ORIENTED_EDGE('',*,*,#21530,.F.);
#31454=ORIENTED_EDGE('',*,*,#21531,.T.);
#31455=ORIENTED_EDGE('',*,*,#21532,.T.);
#31456=ORIENTED_EDGE('',*,*,#21533,.T.);
#31457=ORIENTED_EDGE('',*,*,#21534,.F.);
#31458=ORIENTED_EDGE('',*,*,#21535,.T.);
#31459=ORIENTED_EDGE('',*,*,#21535,.F.);
#31460=ORIENTED_EDGE('',*,*,#21536,.T.);
#31461=ORIENTED_EDGE('',*,*,#21537,.F.);
#31462=ORIENTED_EDGE('',*,*,#21538,.F.);
#31463=ORIENTED_EDGE('',*,*,#21536,.F.);
#31464=ORIENTED_EDGE('',*,*,#21534,.T.);
#31465=ORIENTED_EDGE('',*,*,#21539,.F.);
#31466=ORIENTED_EDGE('',*,*,#21540,.T.);
#31467=ORIENTED_EDGE('',*,*,#21539,.T.);
#31468=ORIENTED_EDGE('',*,*,#21533,.F.);
#31469=ORIENTED_EDGE('',*,*,#21541,.T.);
#31470=ORIENTED_EDGE('',*,*,#21542,.F.);
#31471=ORIENTED_EDGE('',*,*,#21541,.F.);
#31472=ORIENTED_EDGE('',*,*,#21532,.F.);
#31473=ORIENTED_EDGE('',*,*,#21543,.T.);
#31474=ORIENTED_EDGE('',*,*,#21544,.T.);
#31475=ORIENTED_EDGE('',*,*,#21543,.F.);
#31476=ORIENTED_EDGE('',*,*,#21531,.F.);
#31477=ORIENTED_EDGE('',*,*,#21545,.T.);
#31478=ORIENTED_EDGE('',*,*,#21546,.T.);
#31479=ORIENTED_EDGE('',*,*,#21547,.T.);
#31480=ORIENTED_EDGE('',*,*,#21548,.F.);
#31481=ORIENTED_EDGE('',*,*,#21549,.F.);
#31482=ORIENTED_EDGE('',*,*,#21550,.T.);
#31483=ORIENTED_EDGE('',*,*,#21551,.T.);
#31484=ORIENTED_EDGE('',*,*,#21546,.F.);
#31485=ORIENTED_EDGE('',*,*,#21552,.F.);
#31486=ORIENTED_EDGE('',*,*,#21547,.F.);
#31487=ORIENTED_EDGE('',*,*,#21551,.F.);
#31488=ORIENTED_EDGE('',*,*,#21553,.F.);
#31489=ORIENTED_EDGE('',*,*,#21553,.T.);
#31490=ORIENTED_EDGE('',*,*,#21550,.F.);
#31491=ORIENTED_EDGE('',*,*,#21554,.T.);
#31492=ORIENTED_EDGE('',*,*,#21555,.T.);
#31493=ORIENTED_EDGE('',*,*,#21556,.T.);
#31494=ORIENTED_EDGE('',*,*,#21554,.F.);
#31495=ORIENTED_EDGE('',*,*,#21549,.T.);
#31496=ORIENTED_EDGE('',*,*,#21557,.T.);
#31497=ORIENTED_EDGE('',*,*,#21558,.F.);
#31498=ORIENTED_EDGE('',*,*,#21559,.F.);
#31499=ORIENTED_EDGE('',*,*,#21560,.T.);
#31500=ORIENTED_EDGE('',*,*,#21561,.F.);
#31501=ORIENTED_EDGE('',*,*,#21562,.T.);
#31502=ORIENTED_EDGE('',*,*,#21561,.T.);
#31503=ORIENTED_EDGE('',*,*,#21563,.T.);
#31504=ORIENTED_EDGE('',*,*,#21563,.F.);
#31505=ORIENTED_EDGE('',*,*,#21560,.F.);
#31506=ORIENTED_EDGE('',*,*,#21564,.F.);
#31507=ORIENTED_EDGE('',*,*,#21565,.F.);
#31508=ORIENTED_EDGE('',*,*,#21564,.T.);
#31509=ORIENTED_EDGE('',*,*,#21559,.T.);
#31510=ORIENTED_EDGE('',*,*,#21566,.T.);
#31511=ORIENTED_EDGE('',*,*,#21567,.T.);
#31512=ORIENTED_EDGE('',*,*,#21568,.T.);
#31513=ORIENTED_EDGE('',*,*,#21566,.F.);
#31514=ORIENTED_EDGE('',*,*,#21558,.T.);
#31515=ORIENTED_EDGE('',*,*,#21569,.T.);
#31516=ORIENTED_EDGE('',*,*,#21570,.F.);
#31517=ORIENTED_EDGE('',*,*,#21571,.T.);
#31518=ORIENTED_EDGE('',*,*,#21572,.T.);
#31519=ORIENTED_EDGE('',*,*,#21573,.T.);
#31520=ORIENTED_EDGE('',*,*,#21574,.T.);
#31521=ORIENTED_EDGE('',*,*,#21575,.T.);
#31522=ORIENTED_EDGE('',*,*,#21576,.F.);
#31523=ORIENTED_EDGE('',*,*,#21570,.T.);
#31524=ORIENTED_EDGE('',*,*,#21571,.F.);
#31525=ORIENTED_EDGE('',*,*,#21576,.T.);
#31526=ORIENTED_EDGE('',*,*,#21577,.T.);
#31527=ORIENTED_EDGE('',*,*,#21578,.T.);
#31528=ORIENTED_EDGE('',*,*,#21579,.T.);
#31529=ORIENTED_EDGE('',*,*,#21577,.F.);
#31530=ORIENTED_EDGE('',*,*,#21575,.F.);
#31531=ORIENTED_EDGE('',*,*,#21580,.F.);
#31532=ORIENTED_EDGE('',*,*,#21581,.T.);
#31533=ORIENTED_EDGE('',*,*,#21580,.T.);
#31534=ORIENTED_EDGE('',*,*,#21574,.F.);
#31535=ORIENTED_EDGE('',*,*,#21582,.T.);
#31536=ORIENTED_EDGE('',*,*,#21582,.F.);
#31537=ORIENTED_EDGE('',*,*,#21573,.F.);
#31538=ORIENTED_EDGE('',*,*,#21583,.F.);
#31539=ORIENTED_EDGE('',*,*,#21584,.T.);
#31540=ORIENTED_EDGE('',*,*,#21585,.F.);
#31541=ORIENTED_EDGE('',*,*,#21586,.T.);
#31542=ORIENTED_EDGE('',*,*,#21587,.T.);
#31543=ORIENTED_EDGE('',*,*,#21498,.F.);
#31544=ORIENTED_EDGE('',*,*,#21588,.F.);
#31545=ORIENTED_EDGE('',*,*,#21586,.F.);
#31546=ORIENTED_EDGE('',*,*,#21589,.F.);
#31547=ORIENTED_EDGE('',*,*,#21584,.F.);
#31548=ORIENTED_EDGE('',*,*,#21590,.T.);
#31549=ORIENTED_EDGE('',*,*,#21476,.F.);
#31550=ORIENTED_EDGE('',*,*,#21591,.T.);
#31551=ORIENTED_EDGE('',*,*,#21592,.F.);
#31552=ORIENTED_EDGE('',*,*,#21593,.F.);
#31553=ORIENTED_EDGE('',*,*,#21594,.F.);
#31554=ORIENTED_EDGE('',*,*,#21595,.F.);
#31555=ORIENTED_EDGE('',*,*,#21585,.T.);
#31556=ORIENTED_EDGE('',*,*,#21591,.F.);
#31557=ORIENTED_EDGE('',*,*,#21596,.F.);
#31558=ORIENTED_EDGE('',*,*,#21590,.F.);
#31559=ORIENTED_EDGE('',*,*,#21588,.T.);
#31560=ORIENTED_EDGE('',*,*,#21597,.T.);
#31561=ORIENTED_EDGE('',*,*,#21589,.T.);
#31562=ORIENTED_EDGE('',*,*,#21587,.F.);
#31563=ORIENTED_EDGE('',*,*,#21598,.F.);
#31564=ORIENTED_EDGE('',*,*,#21599,.T.);
#31565=ORIENTED_EDGE('',*,*,#21592,.T.);
#31566=ORIENTED_EDGE('',*,*,#21600,.T.);
#31567=ORIENTED_EDGE('',*,*,#21601,.F.);
#31568=ORIENTED_EDGE('',*,*,#21600,.F.);
#31569=ORIENTED_EDGE('',*,*,#21595,.T.);
#31570=ORIENTED_EDGE('',*,*,#21602,.T.);
#31571=ORIENTED_EDGE('',*,*,#21603,.T.);
#31572=ORIENTED_EDGE('',*,*,#21604,.F.);
#31573=ORIENTED_EDGE('',*,*,#21602,.F.);
#31574=ORIENTED_EDGE('',*,*,#21594,.T.);
#31575=ORIENTED_EDGE('',*,*,#21603,.F.);
#31576=ORIENTED_EDGE('',*,*,#21593,.T.);
#31577=ORIENTED_EDGE('',*,*,#21599,.F.);
#31578=ORIENTED_EDGE('',*,*,#21605,.F.);
#31579=ORIENTED_EDGE('',*,*,#21606,.T.);
#31580=ORIENTED_EDGE('',*,*,#21607,.T.);
#31581=ORIENTED_EDGE('',*,*,#21608,.T.);
#31582=ORIENTED_EDGE('',*,*,#21609,.T.);
#31583=ORIENTED_EDGE('',*,*,#21607,.F.);
#31584=ORIENTED_EDGE('',*,*,#21610,.T.);
#31585=ORIENTED_EDGE('',*,*,#21611,.F.);
#31586=ORIENTED_EDGE('',*,*,#21612,.T.);
#31587=ORIENTED_EDGE('',*,*,#21611,.T.);
#31588=ORIENTED_EDGE('',*,*,#21613,.T.);
#31589=ORIENTED_EDGE('',*,*,#21614,.T.);
#31590=ORIENTED_EDGE('',*,*,#21615,.F.);
#31591=ORIENTED_EDGE('',*,*,#21614,.F.);
#31592=ORIENTED_EDGE('',*,*,#21616,.F.);
#31593=ORIENTED_EDGE('',*,*,#21617,.F.);
#31594=ORIENTED_EDGE('',*,*,#21618,.T.);
#31595=ORIENTED_EDGE('',*,*,#21619,.T.);
#31596=ORIENTED_EDGE('',*,*,#21620,.T.);
#31597=ORIENTED_EDGE('',*,*,#21617,.T.);
#31598=ORIENTED_EDGE('',*,*,#21621,.T.);
#31599=ORIENTED_EDGE('',*,*,#21622,.F.);
#31600=ORIENTED_EDGE('',*,*,#21623,.F.);
#31601=ORIENTED_EDGE('',*,*,#21624,.F.);
#31602=ORIENTED_EDGE('',*,*,#21625,.F.);
#31603=ORIENTED_EDGE('',*,*,#21623,.T.);
#31604=ORIENTED_EDGE('',*,*,#21626,.F.);
#31605=ORIENTED_EDGE('',*,*,#21627,.T.);
#31606=ORIENTED_EDGE('',*,*,#21628,.T.);
#31607=ORIENTED_EDGE('',*,*,#21629,.T.);
#31608=ORIENTED_EDGE('',*,*,#21627,.F.);
#31609=ORIENTED_EDGE('',*,*,#21630,.F.);
#31610=ORIENTED_EDGE('',*,*,#21631,.F.);
#31611=ORIENTED_EDGE('',*,*,#21631,.T.);
#31612=ORIENTED_EDGE('',*,*,#21632,.T.);
#31613=ORIENTED_EDGE('',*,*,#21633,.T.);
#31614=ORIENTED_EDGE('',*,*,#21634,.F.);
#31615=ORIENTED_EDGE('',*,*,#21635,.F.);
#31616=ORIENTED_EDGE('',*,*,#21636,.F.);
#31617=ORIENTED_EDGE('',*,*,#21636,.T.);
#31618=ORIENTED_EDGE('',*,*,#21637,.T.);
#31619=ORIENTED_EDGE('',*,*,#21638,.T.);
#31620=ORIENTED_EDGE('',*,*,#21639,.T.);
#31621=ORIENTED_EDGE('',*,*,#21638,.F.);
#31622=ORIENTED_EDGE('',*,*,#21640,.F.);
#31623=ORIENTED_EDGE('',*,*,#21641,.T.);
#31624=ORIENTED_EDGE('',*,*,#21642,.F.);
#31625=ORIENTED_EDGE('',*,*,#21643,.F.);
#31626=ORIENTED_EDGE('',*,*,#21644,.T.);
#31627=ORIENTED_EDGE('',*,*,#21645,.F.);
#31628=ORIENTED_EDGE('',*,*,#21646,.F.);
#31629=ORIENTED_EDGE('',*,*,#21647,.F.);
#31630=ORIENTED_EDGE('',*,*,#21644,.F.);
#31631=ORIENTED_EDGE('',*,*,#21648,.T.);
#31632=ORIENTED_EDGE('',*,*,#21649,.T.);
#31633=ORIENTED_EDGE('',*,*,#21650,.F.);
#31634=ORIENTED_EDGE('',*,*,#21651,.T.);
#31635=ORIENTED_EDGE('',*,*,#21646,.T.);
#31636=ORIENTED_EDGE('',*,*,#21652,.T.);
#31637=ORIENTED_EDGE('',*,*,#21520,.T.);
#31638=ORIENTED_EDGE('',*,*,#21653,.F.);
#31639=ORIENTED_EDGE('',*,*,#21654,.F.);
#31640=ORIENTED_EDGE('',*,*,#21655,.T.);
#31641=ORIENTED_EDGE('',*,*,#21656,.T.);
#31642=ORIENTED_EDGE('',*,*,#21657,.T.);
#31643=ORIENTED_EDGE('',*,*,#21658,.T.);
#31644=ORIENTED_EDGE('',*,*,#21659,.F.);
#31645=ORIENTED_EDGE('',*,*,#21660,.T.);
#31646=ORIENTED_EDGE('',*,*,#21661,.F.);
#31647=ORIENTED_EDGE('',*,*,#21662,.T.);
#31648=ORIENTED_EDGE('',*,*,#21663,.T.);
#31649=ORIENTED_EDGE('',*,*,#21664,.T.);
#31650=ORIENTED_EDGE('',*,*,#21665,.T.);
#31651=ORIENTED_EDGE('',*,*,#21666,.F.);
#31652=ORIENTED_EDGE('',*,*,#21667,.T.);
#31653=ORIENTED_EDGE('',*,*,#21668,.F.);
#31654=ORIENTED_EDGE('',*,*,#21669,.T.);
#31655=ORIENTED_EDGE('',*,*,#21670,.T.);
#31656=ORIENTED_EDGE('',*,*,#21671,.T.);
#31657=ORIENTED_EDGE('',*,*,#21672,.T.);
#31658=ORIENTED_EDGE('',*,*,#21673,.F.);
#31659=ORIENTED_EDGE('',*,*,#21674,.T.);
#31660=ORIENTED_EDGE('',*,*,#21675,.F.);
#31661=ORIENTED_EDGE('',*,*,#21676,.F.);
#31662=ORIENTED_EDGE('',*,*,#21677,.T.);
#31663=ORIENTED_EDGE('',*,*,#21678,.T.);
#31664=ORIENTED_EDGE('',*,*,#21679,.T.);
#31665=ORIENTED_EDGE('',*,*,#21680,.T.);
#31666=ORIENTED_EDGE('',*,*,#21598,.T.);
#31667=ORIENTED_EDGE('',*,*,#21601,.T.);
#31668=ORIENTED_EDGE('',*,*,#21604,.T.);
#31669=ORIENTED_EDGE('',*,*,#21605,.T.);
#31670=ORIENTED_EDGE('',*,*,#21439,.F.);
#31671=ORIENTED_EDGE('',*,*,#21681,.T.);
#31672=ORIENTED_EDGE('',*,*,#21654,.T.);
#31673=ORIENTED_EDGE('',*,*,#21682,.T.);
#31674=ORIENTED_EDGE('',*,*,#21683,.T.);
#31675=ORIENTED_EDGE('',*,*,#21684,.T.);
#31676=ORIENTED_EDGE('',*,*,#21685,.T.);
#31677=ORIENTED_EDGE('',*,*,#21686,.T.);
#31678=ORIENTED_EDGE('',*,*,#21441,.F.);
#31679=ORIENTED_EDGE('',*,*,#21501,.F.);
#31680=ORIENTED_EDGE('',*,*,#21500,.T.);
#31681=ORIENTED_EDGE('',*,*,#21499,.F.);
#31682=ORIENTED_EDGE('',*,*,#21597,.F.);
#31683=ORIENTED_EDGE('',*,*,#21497,.F.);
#31684=ORIENTED_EDGE('',*,*,#21496,.T.);
#31685=ORIENTED_EDGE('',*,*,#21495,.T.);
#31686=ORIENTED_EDGE('',*,*,#21494,.F.);
#31687=ORIENTED_EDGE('',*,*,#21493,.F.);
#31688=ORIENTED_EDGE('',*,*,#21492,.F.);
#31689=ORIENTED_EDGE('',*,*,#21491,.T.);
#31690=ORIENTED_EDGE('',*,*,#21490,.F.);
#31691=ORIENTED_EDGE('',*,*,#21489,.T.);
#31692=ORIENTED_EDGE('',*,*,#21488,.F.);
#31693=ORIENTED_EDGE('',*,*,#21487,.F.);
#31694=ORIENTED_EDGE('',*,*,#21486,.T.);
#31695=ORIENTED_EDGE('',*,*,#21485,.T.);
#31696=ORIENTED_EDGE('',*,*,#21484,.F.);
#31697=ORIENTED_EDGE('',*,*,#21483,.F.);
#31698=ORIENTED_EDGE('',*,*,#21482,.T.);
#31699=ORIENTED_EDGE('',*,*,#21481,.F.);
#31700=ORIENTED_EDGE('',*,*,#21480,.F.);
#31701=ORIENTED_EDGE('',*,*,#21479,.T.);
#31702=ORIENTED_EDGE('',*,*,#21478,.T.);
#31703=ORIENTED_EDGE('',*,*,#21477,.T.);
#31704=ORIENTED_EDGE('',*,*,#21596,.T.);
#31705=ORIENTED_EDGE('',*,*,#21475,.T.);
#31706=ORIENTED_EDGE('',*,*,#21474,.T.);
#31707=ORIENTED_EDGE('',*,*,#21473,.F.);
#31708=ORIENTED_EDGE('',*,*,#21687,.T.);
#31709=ORIENTED_EDGE('',*,*,#21656,.F.);
#31710=ORIENTED_EDGE('',*,*,#21688,.T.);
#31711=ORIENTED_EDGE('',*,*,#21689,.T.);
#31712=ORIENTED_EDGE('',*,*,#21690,.F.);
#31713=ORIENTED_EDGE('',*,*,#21691,.T.);
#31714=ORIENTED_EDGE('',*,*,#21688,.F.);
#31715=ORIENTED_EDGE('',*,*,#21655,.F.);
#31716=ORIENTED_EDGE('',*,*,#21692,.T.);
#31717=ORIENTED_EDGE('',*,*,#21690,.T.);
#31718=ORIENTED_EDGE('',*,*,#21680,.F.);
#31719=ORIENTED_EDGE('',*,*,#21693,.F.);
#31720=ORIENTED_EDGE('',*,*,#21679,.F.);
#31721=ORIENTED_EDGE('',*,*,#21694,.T.);
#31722=ORIENTED_EDGE('',*,*,#21695,.T.);
#31723=ORIENTED_EDGE('',*,*,#21693,.T.);
#31724=ORIENTED_EDGE('',*,*,#21696,.F.);
#31725=ORIENTED_EDGE('',*,*,#21697,.T.);
#31726=ORIENTED_EDGE('',*,*,#21694,.F.);
#31727=ORIENTED_EDGE('',*,*,#21678,.F.);
#31728=ORIENTED_EDGE('',*,*,#21698,.F.);
#31729=ORIENTED_EDGE('',*,*,#21699,.F.);
#31730=ORIENTED_EDGE('',*,*,#21696,.T.);
#31731=ORIENTED_EDGE('',*,*,#21677,.F.);
#31732=ORIENTED_EDGE('',*,*,#21698,.T.);
#31733=ORIENTED_EDGE('',*,*,#21676,.T.);
#31734=ORIENTED_EDGE('',*,*,#21700,.T.);
#31735=ORIENTED_EDGE('',*,*,#21701,.T.);
#31736=ORIENTED_EDGE('',*,*,#21702,.T.);
#31737=ORIENTED_EDGE('',*,*,#21700,.F.);
#31738=ORIENTED_EDGE('',*,*,#21675,.T.);
#31739=ORIENTED_EDGE('',*,*,#21703,.T.);
#31740=ORIENTED_EDGE('',*,*,#21704,.T.);
#31741=ORIENTED_EDGE('',*,*,#21703,.F.);
#31742=ORIENTED_EDGE('',*,*,#21674,.F.);
#31743=ORIENTED_EDGE('',*,*,#21705,.T.);
#31744=ORIENTED_EDGE('',*,*,#21706,.T.);
#31745=ORIENTED_EDGE('',*,*,#21705,.F.);
#31746=ORIENTED_EDGE('',*,*,#21673,.T.);
#31747=ORIENTED_EDGE('',*,*,#21707,.F.);
#31748=ORIENTED_EDGE('',*,*,#21708,.F.);
#31749=ORIENTED_EDGE('',*,*,#21709,.F.);
#31750=ORIENTED_EDGE('',*,*,#21707,.T.);
#31751=ORIENTED_EDGE('',*,*,#21672,.F.);
#31752=ORIENTED_EDGE('',*,*,#21671,.F.);
#31753=ORIENTED_EDGE('',*,*,#21710,.F.);
#31754=ORIENTED_EDGE('',*,*,#21711,.T.);
#31755=ORIENTED_EDGE('',*,*,#21708,.T.);
#31756=ORIENTED_EDGE('',*,*,#21712,.F.);
#31757=ORIENTED_EDGE('',*,*,#21713,.F.);
#31758=ORIENTED_EDGE('',*,*,#21710,.T.);
#31759=ORIENTED_EDGE('',*,*,#21670,.F.);
#31760=ORIENTED_EDGE('',*,*,#21714,.T.);
#31761=ORIENTED_EDGE('',*,*,#21712,.T.);
#31762=ORIENTED_EDGE('',*,*,#21669,.F.);
#31763=ORIENTED_EDGE('',*,*,#21715,.T.);
#31764=ORIENTED_EDGE('',*,*,#21716,.T.);
#31765=ORIENTED_EDGE('',*,*,#21715,.F.);
#31766=ORIENTED_EDGE('',*,*,#21668,.T.);
#31767=ORIENTED_EDGE('',*,*,#21717,.T.);
#31768=ORIENTED_EDGE('',*,*,#21667,.F.);
#31769=ORIENTED_EDGE('',*,*,#21718,.T.);
#31770=ORIENTED_EDGE('',*,*,#21719,.T.);
#31771=ORIENTED_EDGE('',*,*,#21717,.F.);
#31772=ORIENTED_EDGE('',*,*,#21720,.T.);
#31773=ORIENTED_EDGE('',*,*,#21718,.F.);
#31774=ORIENTED_EDGE('',*,*,#21666,.T.);
#31775=ORIENTED_EDGE('',*,*,#21721,.T.);
#31776=ORIENTED_EDGE('',*,*,#21722,.F.);
#31777=ORIENTED_EDGE('',*,*,#21723,.T.);
#31778=ORIENTED_EDGE('',*,*,#21721,.F.);
#31779=ORIENTED_EDGE('',*,*,#21665,.F.);
#31780=ORIENTED_EDGE('',*,*,#21724,.F.);
#31781=ORIENTED_EDGE('',*,*,#21725,.F.);
#31782=ORIENTED_EDGE('',*,*,#21722,.T.);
#31783=ORIENTED_EDGE('',*,*,#21664,.F.);
#31784=ORIENTED_EDGE('',*,*,#21663,.F.);
#31785=ORIENTED_EDGE('',*,*,#21726,.F.);
#31786=ORIENTED_EDGE('',*,*,#21727,.T.);
#31787=ORIENTED_EDGE('',*,*,#21724,.T.);
#31788=ORIENTED_EDGE('',*,*,#21728,.T.);
#31789=ORIENTED_EDGE('',*,*,#21729,.F.);
#31790=ORIENTED_EDGE('',*,*,#21726,.T.);
#31791=ORIENTED_EDGE('',*,*,#21662,.F.);
#31792=ORIENTED_EDGE('',*,*,#21730,.T.);
#31793=ORIENTED_EDGE('',*,*,#21728,.F.);
#31794=ORIENTED_EDGE('',*,*,#21661,.T.);
#31795=ORIENTED_EDGE('',*,*,#21731,.T.);
#31796=ORIENTED_EDGE('',*,*,#21660,.F.);
#31797=ORIENTED_EDGE('',*,*,#21732,.T.);
#31798=ORIENTED_EDGE('',*,*,#21733,.T.);
#31799=ORIENTED_EDGE('',*,*,#21731,.F.);
#31800=ORIENTED_EDGE('',*,*,#21734,.T.);
#31801=ORIENTED_EDGE('',*,*,#21732,.F.);
#31802=ORIENTED_EDGE('',*,*,#21659,.T.);
#31803=ORIENTED_EDGE('',*,*,#21735,.T.);
#31804=ORIENTED_EDGE('',*,*,#21736,.F.);
#31805=ORIENTED_EDGE('',*,*,#21737,.T.);
#31806=ORIENTED_EDGE('',*,*,#21735,.F.);
#31807=ORIENTED_EDGE('',*,*,#21658,.F.);
#31808=ORIENTED_EDGE('',*,*,#21687,.F.);
#31809=ORIENTED_EDGE('',*,*,#21738,.F.);
#31810=ORIENTED_EDGE('',*,*,#21736,.T.);
#31811=ORIENTED_EDGE('',*,*,#21657,.F.);
#31812=ORIENTED_EDGE('',*,*,#21739,.T.);
#31813=ORIENTED_EDGE('',*,*,#21740,.F.);
#31814=ORIENTED_EDGE('',*,*,#21641,.F.);
#31815=ORIENTED_EDGE('',*,*,#21740,.T.);
#31816=ORIENTED_EDGE('',*,*,#21741,.F.);
#31817=ORIENTED_EDGE('',*,*,#21634,.T.);
#31818=ORIENTED_EDGE('',*,*,#21639,.F.);
#31819=ORIENTED_EDGE('',*,*,#21642,.T.);
#31820=ORIENTED_EDGE('',*,*,#21742,.F.);
#31821=ORIENTED_EDGE('',*,*,#21743,.F.);
#31822=ORIENTED_EDGE('',*,*,#21624,.T.);
#31823=ORIENTED_EDGE('',*,*,#21628,.F.);
#31824=ORIENTED_EDGE('',*,*,#21629,.F.);
#31825=ORIENTED_EDGE('',*,*,#21633,.F.);
#31826=ORIENTED_EDGE('',*,*,#21743,.T.);
#31827=ORIENTED_EDGE('',*,*,#21744,.T.);
#31828=ORIENTED_EDGE('',*,*,#21625,.T.);
#31829=ORIENTED_EDGE('',*,*,#21745,.T.);
#31830=ORIENTED_EDGE('',*,*,#21746,.T.);
#31831=ORIENTED_EDGE('',*,*,#21619,.F.);
#31832=ORIENTED_EDGE('',*,*,#21746,.F.);
#31833=ORIENTED_EDGE('',*,*,#21747,.T.);
#31834=ORIENTED_EDGE('',*,*,#21612,.F.);
#31835=ORIENTED_EDGE('',*,*,#21615,.T.);
#31836=ORIENTED_EDGE('',*,*,#21618,.F.);
#31837=ORIENTED_EDGE('',*,*,#21620,.F.);
#31838=ORIENTED_EDGE('',*,*,#21517,.F.);
#31839=ORIENTED_EDGE('',*,*,#21457,.T.);
#31840=ORIENTED_EDGE('',*,*,#21445,.F.);
#31841=ORIENTED_EDGE('',*,*,#21452,.F.);
#31842=ORIENTED_EDGE('',*,*,#21519,.F.);
#31843=ORIENTED_EDGE('',*,*,#21748,.T.);
#31844=ORIENTED_EDGE('',*,*,#21749,.F.);
#31845=ORIENTED_EDGE('',*,*,#21748,.F.);
#31846=ORIENTED_EDGE('',*,*,#21518,.F.);
#31847=ORIENTED_EDGE('',*,*,#21468,.T.);
#31848=ORIENTED_EDGE('',*,*,#21461,.F.);
#31849=ORIENTED_EDGE('',*,*,#21464,.F.);
#31850=ORIENTED_EDGE('',*,*,#21568,.F.);
#31851=ORIENTED_EDGE('',*,*,#21557,.F.);
#31852=ORIENTED_EDGE('',*,*,#21562,.F.);
#31853=ORIENTED_EDGE('',*,*,#21565,.T.);
#31854=ORIENTED_EDGE('',*,*,#21567,.F.);
#31855=ORIENTED_EDGE('',*,*,#21552,.T.);
#31856=ORIENTED_EDGE('',*,*,#21555,.F.);
#31857=ORIENTED_EDGE('',*,*,#21556,.F.);
#31858=ORIENTED_EDGE('',*,*,#21548,.T.);
#31859=ORIENTED_EDGE('',*,*,#21545,.F.);
#31860=ORIENTED_EDGE('',*,*,#21537,.T.);
#31861=ORIENTED_EDGE('',*,*,#21538,.T.);
#31862=ORIENTED_EDGE('',*,*,#21540,.F.);
#31863=ORIENTED_EDGE('',*,*,#21542,.T.);
#31864=ORIENTED_EDGE('',*,*,#21544,.F.);
#31865=ORIENTED_EDGE('',*,*,#21530,.T.);
#31866=ORIENTED_EDGE('',*,*,#21526,.T.);
#31867=ORIENTED_EDGE('',*,*,#21527,.T.);
#31868=ORIENTED_EDGE('',*,*,#21578,.F.);
#31869=ORIENTED_EDGE('',*,*,#21579,.F.);
#31870=ORIENTED_EDGE('',*,*,#21581,.F.);
#31871=ORIENTED_EDGE('',*,*,#21583,.T.);
#31872=ORIENTED_EDGE('',*,*,#21572,.F.);
#31873=ORIENTED_EDGE('',*,*,#21569,.F.);
#31874=ORIENTED_EDGE('',*,*,#21640,.T.);
#31875=ORIENTED_EDGE('',*,*,#21637,.F.);
#31876=ORIENTED_EDGE('',*,*,#21635,.T.);
#31877=ORIENTED_EDGE('',*,*,#21741,.T.);
#31878=ORIENTED_EDGE('',*,*,#21739,.F.);
#31879=ORIENTED_EDGE('',*,*,#21750,.F.);
#31880=ORIENTED_EDGE('',*,*,#21751,.F.);
#31881=ORIENTED_EDGE('',*,*,#21645,.T.);
#31882=ORIENTED_EDGE('',*,*,#21647,.T.);
#31883=ORIENTED_EDGE('',*,*,#21651,.F.);
#31884=ORIENTED_EDGE('',*,*,#21747,.F.);
#31885=ORIENTED_EDGE('',*,*,#21745,.F.);
#31886=ORIENTED_EDGE('',*,*,#21621,.F.);
#31887=ORIENTED_EDGE('',*,*,#21616,.T.);
#31888=ORIENTED_EDGE('',*,*,#21613,.F.);
#31889=ORIENTED_EDGE('',*,*,#21610,.F.);
#31890=ORIENTED_EDGE('',*,*,#21744,.F.);
#31891=ORIENTED_EDGE('',*,*,#21742,.T.);
#31892=ORIENTED_EDGE('',*,*,#21632,.F.);
#31893=ORIENTED_EDGE('',*,*,#21630,.T.);
#31894=ORIENTED_EDGE('',*,*,#21626,.T.);
#31895=ORIENTED_EDGE('',*,*,#21622,.T.);
#31896=ORIENTED_EDGE('',*,*,#21609,.F.);
#31897=ORIENTED_EDGE('',*,*,#21608,.F.);
#31898=ORIENTED_EDGE('',*,*,#21751,.T.);
#31899=ORIENTED_EDGE('',*,*,#21752,.T.);
#31900=ORIENTED_EDGE('',*,*,#21649,.F.);
#31901=ORIENTED_EDGE('',*,*,#21648,.F.);
#31902=ORIENTED_EDGE('',*,*,#21643,.T.);
#31903=ORIENTED_EDGE('',*,*,#21752,.F.);
#31904=ORIENTED_EDGE('',*,*,#21750,.T.);
#31905=ORIENTED_EDGE('',*,*,#21650,.T.);
#31906=ORIENTED_EDGE('',*,*,#21653,.T.);
#31907=ORIENTED_EDGE('',*,*,#21753,.T.);
#31908=ORIENTED_EDGE('',*,*,#21754,.F.);
#31909=ORIENTED_EDGE('',*,*,#21682,.F.);
#31910=ORIENTED_EDGE('',*,*,#21753,.F.);
#31911=ORIENTED_EDGE('',*,*,#21525,.F.);
#31912=ORIENTED_EDGE('',*,*,#21507,.T.);
#31913=ORIENTED_EDGE('',*,*,#21755,.T.);
#31914=ORIENTED_EDGE('',*,*,#21754,.T.);
#31915=ORIENTED_EDGE('',*,*,#21756,.T.);
#31916=ORIENTED_EDGE('',*,*,#21757,.F.);
#31917=ORIENTED_EDGE('',*,*,#21683,.F.);
#31918=ORIENTED_EDGE('',*,*,#21756,.F.);
#31919=ORIENTED_EDGE('',*,*,#21755,.F.);
#31920=ORIENTED_EDGE('',*,*,#21506,.F.);
#31921=ORIENTED_EDGE('',*,*,#21758,.T.);
#31922=ORIENTED_EDGE('',*,*,#21757,.T.);
#31923=ORIENTED_EDGE('',*,*,#21759,.T.);
#31924=ORIENTED_EDGE('',*,*,#21760,.F.);
#31925=ORIENTED_EDGE('',*,*,#21684,.F.);
#31926=ORIENTED_EDGE('',*,*,#21759,.F.);
#31927=ORIENTED_EDGE('',*,*,#21758,.F.);
#31928=ORIENTED_EDGE('',*,*,#21505,.T.);
#31929=ORIENTED_EDGE('',*,*,#21761,.T.);
#31930=ORIENTED_EDGE('',*,*,#21760,.T.);
#31931=ORIENTED_EDGE('',*,*,#21762,.T.);
#31932=ORIENTED_EDGE('',*,*,#21763,.F.);
#31933=ORIENTED_EDGE('',*,*,#21685,.F.);
#31934=ORIENTED_EDGE('',*,*,#21761,.F.);
#31935=ORIENTED_EDGE('',*,*,#21516,.T.);
#31936=ORIENTED_EDGE('',*,*,#21764,.T.);
#31937=ORIENTED_EDGE('',*,*,#21762,.F.);
#31938=ORIENTED_EDGE('',*,*,#21606,.F.);
#31939=ORIENTED_EDGE('',*,*,#21765,.T.);
#31940=ORIENTED_EDGE('',*,*,#21766,.T.);
#31941=ORIENTED_EDGE('',*,*,#21767,.F.);
#31942=ORIENTED_EDGE('',*,*,#21504,.F.);
#31943=ORIENTED_EDGE('',*,*,#21442,.T.);
#31944=ORIENTED_EDGE('',*,*,#21768,.T.);
#31945=ORIENTED_EDGE('',*,*,#21765,.F.);
#31946=ORIENTED_EDGE('',*,*,#21686,.F.);
#31947=ORIENTED_EDGE('',*,*,#21763,.T.);
#31948=ORIENTED_EDGE('',*,*,#21769,.T.);
#31949=ORIENTED_EDGE('',*,*,#21768,.F.);
#31950=ORIENTED_EDGE('',*,*,#21766,.F.);
#31951=ORIENTED_EDGE('',*,*,#21769,.F.);
#31952=ORIENTED_EDGE('',*,*,#21764,.F.);
#31953=ORIENTED_EDGE('',*,*,#21515,.T.);
#31954=ORIENTED_EDGE('',*,*,#21770,.T.);
#31955=ORIENTED_EDGE('',*,*,#21767,.T.);
#31956=ORIENTED_EDGE('',*,*,#21771,.T.);
#31957=ORIENTED_EDGE('',*,*,#21772,.F.);
#31958=ORIENTED_EDGE('',*,*,#21502,.F.);
#31959=ORIENTED_EDGE('',*,*,#21770,.F.);
#31960=ORIENTED_EDGE('',*,*,#21514,.T.);
#31961=ORIENTED_EDGE('',*,*,#21773,.T.);
#31962=ORIENTED_EDGE('',*,*,#21771,.F.);
#31963=ORIENTED_EDGE('',*,*,#21772,.T.);
#31964=ORIENTED_EDGE('',*,*,#21774,.T.);
#31965=ORIENTED_EDGE('',*,*,#21775,.F.);
#31966=ORIENTED_EDGE('',*,*,#21503,.F.);
#31967=ORIENTED_EDGE('',*,*,#21775,.T.);
#31968=ORIENTED_EDGE('',*,*,#21776,.T.);
#31969=ORIENTED_EDGE('',*,*,#21444,.F.);
#31970=ORIENTED_EDGE('',*,*,#21777,.T.);
#31971=ORIENTED_EDGE('',*,*,#21652,.F.);
#31972=ORIENTED_EDGE('',*,*,#21681,.F.);
#31973=ORIENTED_EDGE('',*,*,#21776,.F.);
#31974=ORIENTED_EDGE('',*,*,#21774,.F.);
#31975=ORIENTED_EDGE('',*,*,#21773,.F.);
#31976=ORIENTED_EDGE('',*,*,#21513,.T.);
#31977=ORIENTED_EDGE('',*,*,#21521,.T.);
#31978=ORIENTED_EDGE('',*,*,#21777,.F.);
#31979=ORIENTED_EDGE('',*,*,#21689,.F.);
#31980=ORIENTED_EDGE('',*,*,#21691,.F.);
#31981=ORIENTED_EDGE('',*,*,#21692,.F.);
#31982=ORIENTED_EDGE('',*,*,#21695,.F.);
#31983=ORIENTED_EDGE('',*,*,#21697,.F.);
#31984=ORIENTED_EDGE('',*,*,#21699,.T.);
#31985=ORIENTED_EDGE('',*,*,#21701,.F.);
#31986=ORIENTED_EDGE('',*,*,#21702,.F.);
#31987=ORIENTED_EDGE('',*,*,#21704,.F.);
#31988=ORIENTED_EDGE('',*,*,#21706,.F.);
#31989=ORIENTED_EDGE('',*,*,#21709,.T.);
#31990=ORIENTED_EDGE('',*,*,#21711,.F.);
#31991=ORIENTED_EDGE('',*,*,#21713,.T.);
#31992=ORIENTED_EDGE('',*,*,#21714,.F.);
#31993=ORIENTED_EDGE('',*,*,#21716,.F.);
#31994=ORIENTED_EDGE('',*,*,#21719,.F.);
#31995=ORIENTED_EDGE('',*,*,#21720,.F.);
#31996=ORIENTED_EDGE('',*,*,#21723,.F.);
#31997=ORIENTED_EDGE('',*,*,#21725,.T.);
#31998=ORIENTED_EDGE('',*,*,#21727,.F.);
#31999=ORIENTED_EDGE('',*,*,#21729,.T.);
#32000=ORIENTED_EDGE('',*,*,#21730,.F.);
#32001=ORIENTED_EDGE('',*,*,#21733,.F.);
#32002=ORIENTED_EDGE('',*,*,#21734,.F.);
#32003=ORIENTED_EDGE('',*,*,#21737,.F.);
#32004=ORIENTED_EDGE('',*,*,#21738,.T.);
#32005=ORIENTED_EDGE('',*,*,#21749,.T.);
#32006=ORIENTED_EDGE('',*,*,#21778,.F.);
#32007=ORIENTED_EDGE('',*,*,#21779,.F.);
#32008=ORIENTED_EDGE('',*,*,#21509,.F.);
#32009=ORIENTED_EDGE('',*,*,#21524,.T.);
#32010=ORIENTED_EDGE('',*,*,#21780,.T.);
#32011=ORIENTED_EDGE('',*,*,#21781,.F.);
#32012=ORIENTED_EDGE('',*,*,#21510,.F.);
#32013=ORIENTED_EDGE('',*,*,#21779,.T.);
#32014=ORIENTED_EDGE('',*,*,#21529,.F.);
#32015=ORIENTED_EDGE('',*,*,#21782,.F.);
#32016=ORIENTED_EDGE('',*,*,#21780,.F.);
#32017=ORIENTED_EDGE('',*,*,#21778,.T.);
#32018=ORIENTED_EDGE('',*,*,#21523,.T.);
#32019=ORIENTED_EDGE('',*,*,#21522,.F.);
#32020=ORIENTED_EDGE('',*,*,#21511,.T.);
#32021=ORIENTED_EDGE('',*,*,#21781,.T.);
#32022=ORIENTED_EDGE('',*,*,#21782,.T.);
#34042=ADVANCED_FACE('',(#5294),#443,.T.);
#34043=ADVANCED_FACE('',(#5295),#2452,.T.);
#34044=ADVANCED_FACE('',(#5296),#2453,.F.);
#34045=ADVANCED_FACE('',(#5297),#2454,.F.);
#34046=ADVANCED_FACE('',(#5298),#3234,.F.);
#34047=ADVANCED_FACE('',(#5299),#2455,.F.);
#34048=ADVANCED_FACE('',(#5300),#2456,.T.);
#34049=ADVANCED_FACE('',(#5301),#2457,.F.);
#34050=ADVANCED_FACE('',(#5302),#2458,.F.);
#34051=ADVANCED_FACE('',(#5303),#2459,.F.);
#34052=ADVANCED_FACE('',(#5304),#2460,.T.);
#34053=ADVANCED_FACE('',(#5305),#3235,.F.);
#34054=ADVANCED_FACE('',(#5306,#1316),#2461,.T.);
#34055=ADVANCED_FACE('',(#5307),#859,.F.);
#34056=ADVANCED_FACE('',(#5308),#2462,.T.);
#34057=ADVANCED_FACE('',(#5309),#2463,.F.);
#34058=ADVANCED_FACE('',(#5310),#3236,.F.);
#34059=ADVANCED_FACE('',(#5311),#2464,.F.);
#34060=ADVANCED_FACE('',(#5312),#2465,.T.);
#34061=ADVANCED_FACE('',(#5313),#2466,.T.);
#34062=ADVANCED_FACE('',(#5314),#3237,.T.);
#34063=ADVANCED_FACE('',(#5315),#2467,.F.);
#34064=ADVANCED_FACE('',(#5316),#2468,.T.);
#34065=ADVANCED_FACE('',(#5317),#2469,.T.);
#34066=ADVANCED_FACE('',(#5318),#2470,.F.);
#34067=ADVANCED_FACE('',(#5319),#2471,.F.);
#34068=ADVANCED_FACE('',(#5320),#3238,.T.);
#34069=ADVANCED_FACE('',(#5321),#2472,.F.);
#34070=ADVANCED_FACE('',(#5322),#2473,.F.);
#34071=ADVANCED_FACE('',(#5323),#2474,.F.);
#34072=ADVANCED_FACE('',(#5324),#3239,.T.);
#34073=ADVANCED_FACE('',(#5325),#2475,.T.);
#34074=ADVANCED_FACE('',(#5326),#2476,.T.);
#34075=ADVANCED_FACE('',(#5327),#2477,.T.);
#34076=ADVANCED_FACE('',(#5328),#2478,.F.);
#34077=ADVANCED_FACE('',(#5329),#2479,.T.);
#34078=ADVANCED_FACE('',(#5330),#3240,.T.);
#34079=ADVANCED_FACE('',(#5331),#2480,.F.);
#34080=ADVANCED_FACE('',(#5332),#2481,.T.);
#34081=ADVANCED_FACE('',(#5333),#2482,.F.);
#34082=ADVANCED_FACE('',(#5334),#2483,.F.);
#34083=ADVANCED_FACE('',(#5335),#3241,.F.);
#34084=ADVANCED_FACE('',(#5336),#3242,.F.);
#34085=ADVANCED_FACE('',(#5337),#2484,.T.);
#34086=ADVANCED_FACE('',(#5338),#2485,.T.);
#34087=ADVANCED_FACE('',(#5339),#2486,.F.);
#34088=ADVANCED_FACE('',(#5340),#3243,.F.);
#34089=ADVANCED_FACE('',(#5341),#3244,.T.);
#34090=ADVANCED_FACE('',(#5342),#2487,.T.);
#34091=ADVANCED_FACE('',(#5343),#3245,.T.);
#34092=ADVANCED_FACE('',(#5344),#3246,.F.);
#34093=ADVANCED_FACE('',(#5345),#2488,.T.);
#34094=ADVANCED_FACE('',(#5346),#2489,.T.);
#34095=ADVANCED_FACE('',(#5347),#3247,.T.);
#34096=ADVANCED_FACE('',(#5348),#2490,.F.);
#34097=ADVANCED_FACE('',(#5349),#2491,.T.);
#34098=ADVANCED_FACE('',(#5350),#3248,.T.);
#34099=ADVANCED_FACE('',(#5351),#2492,.F.);
#34100=ADVANCED_FACE('',(#5352),#2493,.T.);
#34101=ADVANCED_FACE('',(#5353),#2494,.F.);
#34102=ADVANCED_FACE('',(#5354),#3249,.T.);
#34103=ADVANCED_FACE('',(#5355),#2495,.T.);
#34104=ADVANCED_FACE('',(#5356),#2496,.F.);
#34105=ADVANCED_FACE('',(#5357),#3250,.T.);
#34106=ADVANCED_FACE('',(#5358),#2497,.F.);
#34107=ADVANCED_FACE('',(#5359),#3251,.T.);
#34108=ADVANCED_FACE('',(#5360,#1317,#1318),#2498,.F.);
#34109=ADVANCED_FACE('',(#5361),#3252,.T.);
#34110=ADVANCED_FACE('',(#5362),#2499,.F.);
#34111=ADVANCED_FACE('',(#5363),#3253,.T.);
#34112=ADVANCED_FACE('',(#5364),#2500,.F.);
#34113=ADVANCED_FACE('',(#5365),#3254,.T.);
#34114=ADVANCED_FACE('',(#5366),#3255,.F.);
#34115=ADVANCED_FACE('',(#5367),#2501,.T.);
#34116=ADVANCED_FACE('',(#5368),#3256,.T.);
#34117=ADVANCED_FACE('',(#5369),#3257,.T.);
#34118=ADVANCED_FACE('',(#5370),#3258,.T.);
#34119=ADVANCED_FACE('',(#5371),#3259,.F.);
#34120=ADVANCED_FACE('',(#5372),#3260,.T.);
#34121=ADVANCED_FACE('',(#5373),#3261,.F.);
#34122=ADVANCED_FACE('',(#5374),#2502,.T.);
#34123=ADVANCED_FACE('',(#5375),#3262,.T.);
#34124=ADVANCED_FACE('',(#5376),#3263,.T.);
#34125=ADVANCED_FACE('',(#5377),#3264,.T.);
#34126=ADVANCED_FACE('',(#5378),#2503,.F.);
#34127=ADVANCED_FACE('',(#5379),#3265,.F.);
#34128=ADVANCED_FACE('',(#5380),#3266,.T.);
#34129=ADVANCED_FACE('',(#5381),#3267,.F.);
#34130=ADVANCED_FACE('',(#5382),#3268,.T.);
#34131=ADVANCED_FACE('',(#5383),#3269,.T.);
#34132=ADVANCED_FACE('',(#5384),#3270,.T.);
#34133=ADVANCED_FACE('',(#5385),#2504,.F.);
#34134=ADVANCED_FACE('',(#5386),#3271,.F.);
#34135=ADVANCED_FACE('',(#5387),#2505,.T.);
#34136=ADVANCED_FACE('',(#5388),#2506,.T.);
#34137=ADVANCED_FACE('',(#5389),#2507,.T.);
#34138=ADVANCED_FACE('',(#5390),#2508,.T.);
#34139=ADVANCED_FACE('',(#5391),#2509,.T.);
#34140=ADVANCED_FACE('',(#5392),#2510,.T.);
#34141=ADVANCED_FACE('',(#5393,#1319,#1320,#1321,#1322,#1323,#1324,#1325,
#1326,#1327,#1328),#3272,.T.);
#34142=ADVANCED_FACE('',(#5394),#2511,.T.);
#34143=ADVANCED_FACE('',(#5395),#2512,.T.);
#34144=ADVANCED_FACE('',(#5396),#444,.T.);
#34145=ADVANCED_FACE('',(#5397),#3273,.F.);
#34146=ADVANCED_FACE('',(#5398),#3274,.T.);
#34147=ADVANCED_FACE('',(#5399),#2513,.F.);
#34148=ADVANCED_FACE('',(#5400),#445,.T.);
#34149=ADVANCED_FACE('',(#5401),#3275,.F.);
#34150=ADVANCED_FACE('',(#5402),#3276,.T.);
#34151=ADVANCED_FACE('',(#5403,#1329),#2514,.T.);
#34152=ADVANCED_FACE('',(#5404),#1252,.F.);
#34153=ADVANCED_FACE('',(#5405),#860,.T.);
#34154=ADVANCED_FACE('',(#5406),#446,.T.);
#34155=ADVANCED_FACE('',(#5407),#3277,.F.);
#34156=ADVANCED_FACE('',(#5408),#447,.T.);
#34157=ADVANCED_FACE('',(#5409),#2515,.T.);
#34158=ADVANCED_FACE('',(#5410),#1253,.F.);
#34159=ADVANCED_FACE('',(#5411),#861,.T.);
#34160=ADVANCED_FACE('',(#5412),#448,.T.);
#34161=ADVANCED_FACE('',(#5413),#3278,.F.);
#34162=ADVANCED_FACE('',(#5414,#1330),#2516,.F.);
#34163=ADVANCED_FACE('',(#5415),#2517,.T.);
#34164=ADVANCED_FACE('',(#5416,#1331),#2518,.T.);
#34165=ADVANCED_FACE('',(#5417),#2519,.T.);
#34166=ADVANCED_FACE('',(#5418),#2520,.F.);
#34178=CLOSED_SHELL('',(#34042,#34043,#34044,#34045,#34046,#34047,#34048,
#34049,#34050,#34051,#34052,#34053,#34054,#34055,#34056,#34057,#34058,#34059,
#34060,#34061,#34062,#34063,#34064,#34065,#34066,#34067,#34068,#34069,#34070,
#34071,#34072,#34073,#34074,#34075,#34076,#34077,#34078,#34079,#34080,#34081,
#34082,#34083,#34084,#34085,#34086,#34087,#34088,#34089,#34090,#34091,#34092,
#34093,#34094,#34095,#34096,#34097,#34098,#34099,#34100,#34101,#34102,#34103,
#34104,#34105,#34106,#34107,#34108,#34109,#34110,#34111,#34112,#34113,#34114,
#34115,#34116,#34117,#34118,#34119,#34120,#34121,#34122,#34123,#34124,#34125,
#34126,#34127,#34128,#34129,#34130,#34131,#34132,#34133,#34134,#34135,#34136,
#34137,#34138,#34139,#34140,#34141,#34142,#34143,#34144,#34145,#34146,#34147,
#34148,#34149,#34150,#34151,#34152,#34153,#34154,#34155,#34156,#34157,#34158,
#34159,#34160,#34161,#34162,#34163,#34164,#34165,#34166));
#38347=AXIS2_PLACEMENT_3D('',#97330,#48377,#48378);
#38348=AXIS2_PLACEMENT_3D('',#97331,#48379,#48380);
#38349=AXIS2_PLACEMENT_3D('',#97334,#48381,#48382);
#38350=AXIS2_PLACEMENT_3D('',#97336,#48383,#48384);
#38351=AXIS2_PLACEMENT_3D('',#97338,#48385,#48386);
#38352=AXIS2_PLACEMENT_3D('',#97340,#48387,#48388);
#38353=AXIS2_PLACEMENT_3D('',#97342,#48389,#48390);
#38354=AXIS2_PLACEMENT_3D('',#97343,#48391,#48392);
#38355=AXIS2_PLACEMENT_3D('',#97344,#48393,#48394);
#38356=AXIS2_PLACEMENT_3D('',#97347,#48395,#48396);
#38357=AXIS2_PLACEMENT_3D('',#97351,#48398,#48399);
#38358=AXIS2_PLACEMENT_3D('',#97355,#48402,#48403);
#38359=AXIS2_PLACEMENT_3D('',#97361,#48407,#48408);
#38360=AXIS2_PLACEMENT_3D('',#97365,#48411,#48412);
#38361=AXIS2_PLACEMENT_3D('',#97368,#48414,#48415);
#38362=AXIS2_PLACEMENT_3D('',#97369,#48416,#48417);
#38363=AXIS2_PLACEMENT_3D('',#97373,#48420,#48421);
#38364=AXIS2_PLACEMENT_3D('',#97380,#48424,#48425);
#38365=AXIS2_PLACEMENT_3D('',#97382,#48427,#48428);
#38366=AXIS2_PLACEMENT_3D('',#97388,#48432,#48433);
#38367=AXIS2_PLACEMENT_3D('',#97392,#48436,#48437);
#38368=AXIS2_PLACEMENT_3D('',#97396,#48440,#48441);
#38369=AXIS2_PLACEMENT_3D('',#97398,#48442,#48443);
#38370=AXIS2_PLACEMENT_3D('',#97399,#48444,#48445);
#38371=AXIS2_PLACEMENT_3D('',#97402,#48447,#48448);
#38372=AXIS2_PLACEMENT_3D('',#97403,#48449,#48450);
#38373=AXIS2_PLACEMENT_3D('',#97407,#48452,#48453);
#38374=AXIS2_PLACEMENT_3D('',#97411,#48455,#48456);
#38375=AXIS2_PLACEMENT_3D('',#97415,#48458,#48459);
#38376=AXIS2_PLACEMENT_3D('',#97417,#48460,#48461);
#38377=AXIS2_PLACEMENT_3D('',#97421,#48463,#48464);
#38378=AXIS2_PLACEMENT_3D('',#97423,#48465,#48466);
#38379=AXIS2_PLACEMENT_3D('',#97427,#48468,#48469);
#38380=AXIS2_PLACEMENT_3D('',#97429,#48470,#48471);
#38381=AXIS2_PLACEMENT_3D('',#97431,#48472,#48473);
#38382=AXIS2_PLACEMENT_3D('',#97433,#48474,#48475);
#38383=AXIS2_PLACEMENT_3D('',#97435,#48476,#48477);
#38384=AXIS2_PLACEMENT_3D('',#97437,#48478,#48479);
#38385=AXIS2_PLACEMENT_3D('',#97439,#48480,#48481);
#38386=AXIS2_PLACEMENT_3D('',#97443,#48483,#48484);
#38387=AXIS2_PLACEMENT_3D('',#97445,#48485,#48486);
#38388=AXIS2_PLACEMENT_3D('',#97449,#48488,#48489);
#38389=AXIS2_PLACEMENT_3D('',#97451,#48490,#48491);
#38390=AXIS2_PLACEMENT_3D('',#97455,#48493,#48494);
#38391=AXIS2_PLACEMENT_3D('',#97459,#48496,#48497);
#38392=AXIS2_PLACEMENT_3D('',#97461,#48499,#48500);
#38393=AXIS2_PLACEMENT_3D('',#97464,#48501,#48502);
#38394=AXIS2_PLACEMENT_3D('',#97478,#48503,#48504);
#38395=AXIS2_PLACEMENT_3D('',#97480,#48505,#48506);
#38396=AXIS2_PLACEMENT_3D('',#97484,#48508,#48509);
#38397=AXIS2_PLACEMENT_3D('',#97496,#48515,#48516);
#38398=AXIS2_PLACEMENT_3D('',#97500,#48518,#48519);
#38399=AXIS2_PLACEMENT_3D('',#97502,#48521,#48522);
#38400=AXIS2_PLACEMENT_3D('',#97504,#48523,#48524);
#38401=AXIS2_PLACEMENT_3D('',#97505,#48525,#48526);
#38402=AXIS2_PLACEMENT_3D('',#97506,#48527,#48528);
#38403=AXIS2_PLACEMENT_3D('',#97517,#48535,#48536);
#38404=AXIS2_PLACEMENT_3D('',#97559,#48538,#48539);
#38405=AXIS2_PLACEMENT_3D('',#97560,#48540,#48541);
#38406=AXIS2_PLACEMENT_3D('',#97569,#48545,#48546);
#38407=AXIS2_PLACEMENT_3D('',#97573,#48549,#48550);
#38408=AXIS2_PLACEMENT_3D('',#97576,#48552,#48553);
#38409=AXIS2_PLACEMENT_3D('',#97577,#48554,#48555);
#38410=AXIS2_PLACEMENT_3D('',#97581,#48558,#48559);
#38411=AXIS2_PLACEMENT_3D('',#97594,#48561,#48562);
#38412=AXIS2_PLACEMENT_3D('',#97598,#48565,#48566);
#38413=AXIS2_PLACEMENT_3D('',#97599,#48567,#48568);
#38414=AXIS2_PLACEMENT_3D('',#97600,#48569,#48570);
#38415=AXIS2_PLACEMENT_3D('',#97603,#48571,#48572);
#38416=AXIS2_PLACEMENT_3D('',#97607,#48575,#48576);
#38417=AXIS2_PLACEMENT_3D('',#97613,#48579,#48580);
#38418=AXIS2_PLACEMENT_3D('',#97615,#48582,#48583);
#38419=AXIS2_PLACEMENT_3D('',#97619,#48586,#48587);
#38420=AXIS2_PLACEMENT_3D('',#97632,#48589,#48590);
#38421=AXIS2_PLACEMENT_3D('',#97633,#48591,#48592);
#38422=AXIS2_PLACEMENT_3D('',#97634,#48593,#48594);
#38423=AXIS2_PLACEMENT_3D('',#97643,#48598,#48599);
#38424=AXIS2_PLACEMENT_3D('',#97645,#48601,#48602);
#38425=AXIS2_PLACEMENT_3D('',#97647,#48603,#48604);
#38426=AXIS2_PLACEMENT_3D('',#97649,#48606,#48607);
#38427=AXIS2_PLACEMENT_3D('',#97662,#48609,#48610);
#38428=AXIS2_PLACEMENT_3D('',#97666,#48613,#48614);
#38429=AXIS2_PLACEMENT_3D('',#97667,#48615,#48616);
#38430=AXIS2_PLACEMENT_3D('',#97668,#48617,#48618);
#38431=AXIS2_PLACEMENT_3D('',#97671,#48619,#48620);
#38432=AXIS2_PLACEMENT_3D('',#97675,#48623,#48624);
#38433=AXIS2_PLACEMENT_3D('',#97683,#48628,#48629);
#38434=AXIS2_PLACEMENT_3D('',#97685,#48631,#48632);
#38435=AXIS2_PLACEMENT_3D('',#97689,#48635,#48636);
#38436=AXIS2_PLACEMENT_3D('',#97702,#48638,#48639);
#38437=AXIS2_PLACEMENT_3D('',#97706,#48642,#48643);
#38438=AXIS2_PLACEMENT_3D('',#97707,#48644,#48645);
#38439=AXIS2_PLACEMENT_3D('',#97708,#48646,#48647);
#38440=AXIS2_PLACEMENT_3D('',#97711,#48648,#48649);
#38441=AXIS2_PLACEMENT_3D('',#97713,#48651,#48652);
#38442=AXIS2_PLACEMENT_3D('',#97716,#48653,#48654);
#38443=AXIS2_PLACEMENT_3D('',#97718,#48656,#48657);
#38444=AXIS2_PLACEMENT_3D('',#97721,#48660,#48661);
#38445=AXIS2_PLACEMENT_3D('',#97724,#48664,#48665);
#38446=AXIS2_PLACEMENT_3D('',#97727,#48666,#48667);
#38447=AXIS2_PLACEMENT_3D('',#97729,#48668,#48669);
#38448=AXIS2_PLACEMENT_3D('',#97732,#48671,#48672);
#38449=AXIS2_PLACEMENT_3D('',#97733,#48673,#48674);
#38450=AXIS2_PLACEMENT_3D('',#97735,#48676,#48677);
#38451=AXIS2_PLACEMENT_3D('',#97737,#48679,#48680);
#38452=AXIS2_PLACEMENT_3D('',#97740,#48681,#48682);
#38453=AXIS2_PLACEMENT_3D('',#97743,#48685,#48686);
#38454=AXIS2_PLACEMENT_3D('',#97745,#48687,#48688);
#38455=AXIS2_PLACEMENT_3D('',#97747,#48690,#48691);
#38456=AXIS2_PLACEMENT_3D('',#97751,#48694,#48695);
#38457=AXIS2_PLACEMENT_3D('',#97752,#48696,#48697);
#38458=AXIS2_PLACEMENT_3D('',#97753,#48698,#48699);
#38459=AXIS2_PLACEMENT_3D('',#97755,#48700,#48701);
#38460=AXIS2_PLACEMENT_3D('',#97796,#48703,#48704);
#38461=AXIS2_PLACEMENT_3D('',#97799,#48705,#48706);
#38462=AXIS2_PLACEMENT_3D('',#97803,#48709,#48710);
#38463=AXIS2_PLACEMENT_3D('',#97809,#48714,#48715);
#38464=AXIS2_PLACEMENT_3D('',#97823,#48717,#48718);
#38465=AXIS2_PLACEMENT_3D('',#97824,#48719,#48720);
#38466=AXIS2_PLACEMENT_3D('',#97830,#48724,#48725);
#38467=AXIS2_PLACEMENT_3D('',#97839,#48730,#48731);
#38468=AXIS2_PLACEMENT_3D('',#97853,#48733,#48734);
#38469=AXIS2_PLACEMENT_3D('',#97854,#48735,#48736);
#38470=AXIS2_PLACEMENT_3D('',#97860,#48740,#48741);
#38471=AXIS2_PLACEMENT_3D('',#97862,#48742,#48743);
#38472=AXIS2_PLACEMENT_3D('',#97864,#48745,#48746);
#38473=AXIS2_PLACEMENT_3D('',#97869,#48748,#48749);
#38474=AXIS2_PLACEMENT_3D('',#97871,#48751,#48752);
#38475=AXIS2_PLACEMENT_3D('',#97885,#48754,#48755);
#38476=AXIS2_PLACEMENT_3D('',#97886,#48756,#48757);
#38477=AXIS2_PLACEMENT_3D('',#97892,#48761,#48762);
#38478=AXIS2_PLACEMENT_3D('',#97898,#48765,#48766);
#38479=AXIS2_PLACEMENT_3D('',#97899,#48767,#48768);
#38480=AXIS2_PLACEMENT_3D('',#97913,#48770,#48771);
#38481=AXIS2_PLACEMENT_3D('',#97914,#48772,#48773);
#38482=AXIS2_PLACEMENT_3D('',#97920,#48777,#48778);
#38483=AXIS2_PLACEMENT_3D('',#97922,#48779,#48780);
#38484=AXIS2_PLACEMENT_3D('',#97924,#48781,#48782);
#38485=AXIS2_PLACEMENT_3D('',#97926,#48784,#48785);
#38486=AXIS2_PLACEMENT_3D('',#97931,#48787,#48788);
#38487=AXIS2_PLACEMENT_3D('',#97933,#48789,#48790);
#38488=AXIS2_PLACEMENT_3D('',#97937,#48792,#48793);
#38489=AXIS2_PLACEMENT_3D('',#97939,#48794,#48795);
#38490=AXIS2_PLACEMENT_3D('',#97941,#48796,#48797);
#38491=AXIS2_PLACEMENT_3D('',#97943,#48798,#48799);
#38492=AXIS2_PLACEMENT_3D('',#97945,#48800,#48801);
#38493=AXIS2_PLACEMENT_3D('',#97947,#48802,#48803);
#38494=AXIS2_PLACEMENT_3D('',#97951,#48805,#48806);
#38495=AXIS2_PLACEMENT_3D('',#97953,#48807,#48808);
#38496=AXIS2_PLACEMENT_3D('',#97955,#48809,#48810);
#38497=AXIS2_PLACEMENT_3D('',#97959,#48812,#48813);
#38498=AXIS2_PLACEMENT_3D('',#97961,#48814,#48815);
#38499=AXIS2_PLACEMENT_3D('',#97963,#48816,#48817);
#38500=AXIS2_PLACEMENT_3D('',#97965,#48818,#48819);
#38501=AXIS2_PLACEMENT_3D('',#97967,#48820,#48821);
#38502=AXIS2_PLACEMENT_3D('',#97969,#48822,#48823);
#38503=AXIS2_PLACEMENT_3D('',#97973,#48825,#48826);
#38504=AXIS2_PLACEMENT_3D('',#97975,#48827,#48828);
#38505=AXIS2_PLACEMENT_3D('',#97978,#48830,#48831);
#38506=AXIS2_PLACEMENT_3D('',#97979,#48832,#48833);
#38507=AXIS2_PLACEMENT_3D('',#97981,#48834,#48835);
#38508=AXIS2_PLACEMENT_3D('',#97985,#48837,#48838);
#38509=AXIS2_PLACEMENT_3D('',#97988,#48840,#48841);
#38510=AXIS2_PLACEMENT_3D('',#97989,#48842,#48843);
#38511=AXIS2_PLACEMENT_3D('',#97994,#48846,#48847);
#38512=AXIS2_PLACEMENT_3D('',#97995,#48848,#48849);
#38513=AXIS2_PLACEMENT_3D('',#97999,#48852,#48853);
#38514=AXIS2_PLACEMENT_3D('',#98001,#48854,#48855);
#38515=AXIS2_PLACEMENT_3D('',#98003,#48857,#48858);
#38516=AXIS2_PLACEMENT_3D('',#98007,#48861,#48862);
#38517=AXIS2_PLACEMENT_3D('',#98010,#48864,#48865);
#38518=AXIS2_PLACEMENT_3D('',#98011,#48866,#48867);
#38519=AXIS2_PLACEMENT_3D('',#98014,#48869,#48870);
#38520=AXIS2_PLACEMENT_3D('',#98015,#48871,#48872);
#38521=AXIS2_PLACEMENT_3D('',#98019,#48875,#48876);
#38522=AXIS2_PLACEMENT_3D('',#98021,#48877,#48878);
#38523=AXIS2_PLACEMENT_3D('',#98023,#48880,#48881);
#38524=AXIS2_PLACEMENT_3D('',#98025,#48882,#48883);
#38525=AXIS2_PLACEMENT_3D('',#98027,#48885,#48886);
#38526=AXIS2_PLACEMENT_3D('',#98029,#48887,#48888);
#38527=AXIS2_PLACEMENT_3D('',#98031,#48890,#48891);
#38528=AXIS2_PLACEMENT_3D('',#98034,#48893,#48894);
#38529=AXIS2_PLACEMENT_3D('',#98035,#48895,#48896);
#38530=AXIS2_PLACEMENT_3D('',#98038,#48898,#48899);
#38531=AXIS2_PLACEMENT_3D('',#98039,#48900,#48901);
#38532=AXIS2_PLACEMENT_3D('',#98042,#48903,#48904);
#38533=AXIS2_PLACEMENT_3D('',#98043,#48905,#48906);
#38534=AXIS2_PLACEMENT_3D('',#98047,#48909,#48910);
#38535=AXIS2_PLACEMENT_3D('',#98049,#48911,#48912);
#38536=AXIS2_PLACEMENT_3D('',#98051,#48914,#48915);
#38537=AXIS2_PLACEMENT_3D('',#98054,#48917,#48918);
#38538=AXIS2_PLACEMENT_3D('',#98055,#48919,#48920);
#38539=AXIS2_PLACEMENT_3D('',#98057,#48921,#48922);
#38540=AXIS2_PLACEMENT_3D('',#98059,#48924,#48925);
#38541=AXIS2_PLACEMENT_3D('',#98063,#48928,#48929);
#38542=AXIS2_PLACEMENT_3D('',#98066,#48931,#48932);
#38543=AXIS2_PLACEMENT_3D('',#98067,#48933,#48934);
#38544=AXIS2_PLACEMENT_3D('',#98070,#48936,#48937);
#38545=AXIS2_PLACEMENT_3D('',#98071,#48938,#48939);
#38546=AXIS2_PLACEMENT_3D('',#98074,#48941,#48942);
#38547=AXIS2_PLACEMENT_3D('',#98075,#48943,#48944);
#38548=AXIS2_PLACEMENT_3D('',#98077,#48945,#48946);
#38549=AXIS2_PLACEMENT_3D('',#98079,#48948,#48949);
#38550=AXIS2_PLACEMENT_3D('',#98082,#48951,#48952);
#38551=AXIS2_PLACEMENT_3D('',#98083,#48953,#48954);
#38552=AXIS2_PLACEMENT_3D('',#98085,#48955,#48956);
#38553=AXIS2_PLACEMENT_3D('',#98087,#48958,#48959);
#38554=AXIS2_PLACEMENT_3D('',#98091,#48962,#48963);
#38555=AXIS2_PLACEMENT_3D('',#98092,#48964,#48965);
#38556=AXIS2_PLACEMENT_3D('',#98093,#48966,#48967);
#38557=AXIS2_PLACEMENT_3D('',#98095,#48968,#48969);
#38558=AXIS2_PLACEMENT_3D('',#98097,#48971,#48972);
#38559=AXIS2_PLACEMENT_3D('',#98099,#48974,#48975);
#38560=AXIS2_PLACEMENT_3D('',#98103,#48978,#48979);
#38561=AXIS2_PLACEMENT_3D('',#98104,#48980,#48981);
#38562=AXIS2_PLACEMENT_3D('',#98105,#48982,#48983);
#38563=AXIS2_PLACEMENT_3D('',#98107,#48984,#48985);
#38564=AXIS2_PLACEMENT_3D('',#98109,#48987,#48988);
#38565=AXIS2_PLACEMENT_3D('',#98111,#48990,#48991);
#38566=AXIS2_PLACEMENT_3D('',#98114,#48993,#48994);
#38567=AXIS2_PLACEMENT_3D('',#98116,#48995,#48996);
#38568=AXIS2_PLACEMENT_3D('',#98118,#48998,#48999);
#38569=AXIS2_PLACEMENT_3D('',#98120,#49001,#49002);
#38570=AXIS2_PLACEMENT_3D('',#98121,#49003,#49004);
#38571=AXIS2_PLACEMENT_3D('',#98123,#49005,#49006);
#38572=AXIS2_PLACEMENT_3D('',#98124,#49007,#49008);
#38573=AXIS2_PLACEMENT_3D('',#98125,#49009,#49010);
#38574=AXIS2_PLACEMENT_3D('',#98127,#49012,#49013);
#38575=AXIS2_PLACEMENT_3D('',#98130,#49015,#49016);
#38576=AXIS2_PLACEMENT_3D('',#98131,#49017,#49018);
#38577=AXIS2_PLACEMENT_3D('',#98133,#49020,#49021);
#38578=AXIS2_PLACEMENT_3D('',#98135,#49022,#49023);
#38579=AXIS2_PLACEMENT_3D('',#98136,#49024,#49025);
#38580=AXIS2_PLACEMENT_3D('',#98137,#49026,#49027);
#38581=AXIS2_PLACEMENT_3D('',#98139,#49029,#49030);
#38582=AXIS2_PLACEMENT_3D('',#98142,#49032,#49033);
#38583=AXIS2_PLACEMENT_3D('',#98143,#49034,#49035);
#38584=AXIS2_PLACEMENT_3D('',#98182,#49037,#49038);
#38585=AXIS2_PLACEMENT_3D('',#98194,#49039,#49040);
#38586=AXIS2_PLACEMENT_3D('',#98195,#49041,#49042);
#38587=AXIS2_PLACEMENT_3D('',#98196,#49043,#49044);
#38588=AXIS2_PLACEMENT_3D('',#98197,#49045,#49046);
#38589=AXIS2_PLACEMENT_3D('',#98198,#49047,#49048);
#38590=AXIS2_PLACEMENT_3D('',#98199,#49049,#49050);
#38591=AXIS2_PLACEMENT_3D('',#98201,#49052,#49053);
#38592=AXIS2_PLACEMENT_3D('',#98203,#49054,#49055);
#38593=AXIS2_PLACEMENT_3D('',#98204,#49056,#49057);
#38594=AXIS2_PLACEMENT_3D('',#98205,#49058,#49059);
#38595=AXIS2_PLACEMENT_3D('',#98251,#49061,#49062);
#38596=AXIS2_PLACEMENT_3D('',#98252,#49063,#49064);
#38597=AXIS2_PLACEMENT_3D('',#98253,#49065,#49066);
#38598=AXIS2_PLACEMENT_3D('',#98254,#49067,#49068);
#38599=AXIS2_PLACEMENT_3D('',#98255,#49069,#49070);
#38600=AXIS2_PLACEMENT_3D('',#98256,#49071,#49072);
#38601=AXIS2_PLACEMENT_3D('',#98257,#49073,#49074);
#38602=AXIS2_PLACEMENT_3D('',#98258,#49075,#49076);
#38603=AXIS2_PLACEMENT_3D('',#98262,#49079,#49080);
#38604=AXIS2_PLACEMENT_3D('',#98266,#49083,#49084);
#38605=AXIS2_PLACEMENT_3D('',#98268,#49086,#49087);
#48377=DIRECTION('axis',(0.,0.,1.));
#48378=DIRECTION('refdir',(1.,0.,0.));
#48379=DIRECTION('center_axis',(0.,-1.,0.));
#48380=DIRECTION('ref_axis',(-0.864870204545057,0.,-0.501995547082034));
#48381=DIRECTION('center_axis',(0.,-1.,0.));
#48382=DIRECTION('ref_axis',(1.,0.,0.));
#48383=DIRECTION('center_axis',(0.,-1.,0.));
#48384=DIRECTION('ref_axis',(1.,0.,0.));
#48385=DIRECTION('center_axis',(0.,-1.,0.));
#48386=DIRECTION('ref_axis',(1.,0.,0.));
#48387=DIRECTION('center_axis',(0.362576028100137,-1.34614541736051E-15,
0.931954196217351));
#48388=DIRECTION('ref_axis',(0.931954196217351,6.44102416595859E-31,-0.362576028100137));
#48389=DIRECTION('center_axis',(0.,-1.,0.));
#48390=DIRECTION('ref_axis',(1.,0.,0.));
#48391=DIRECTION('center_axis',(0.362576028100137,-9.99200722163376E-16,
-0.931954196217351));
#48392=DIRECTION('ref_axis',(0.931954196217351,4.30399528931578E-31,0.362576028100137));
#48393=DIRECTION('center_axis',(0.,1.,0.));
#48394=DIRECTION('ref_axis',(1.,0.,0.));
#48395=DIRECTION('center_axis',(0.,1.,0.));
#48396=DIRECTION('ref_axis',(1.,0.,0.));
#48397=DIRECTION('',(-0.838443593764828,0.,-0.544988385265888));
#48398=DIRECTION('center_axis',(0.,-1.,0.));
#48399=DIRECTION('ref_axis',(1.,0.,0.));
#48400=DIRECTION('',(0.,0.,1.));
#48401=DIRECTION('',(0.612862105001227,0.,0.790189876076292));
#48402=DIRECTION('center_axis',(0.790189876076292,0.,-0.612862105001227));
#48403=DIRECTION('ref_axis',(0.,-1.,0.));
#48404=DIRECTION('',(0.,1.,0.));
#48405=DIRECTION('',(0.612862105001227,0.,0.790189876076292));
#48406=DIRECTION('',(0.,1.,0.));
#48407=DIRECTION('center_axis',(1.,0.,0.));
#48408=DIRECTION('ref_axis',(0.,1.,0.));
#48409=DIRECTION('',(0.,1.,0.));
#48410=DIRECTION('',(0.,0.,1.));
#48411=DIRECTION('center_axis',(0.,1.,0.));
#48412=DIRECTION('ref_axis',(0.617975203688407,0.,0.786197588158519));
#48413=DIRECTION('',(0.,1.,0.));
#48414=DIRECTION('center_axis',(0.,-1.,0.));
#48415=DIRECTION('ref_axis',(1.,0.,0.));
#48416=DIRECTION('center_axis',(-0.544988385265888,0.,0.838443593764828));
#48417=DIRECTION('ref_axis',(0.,1.,0.));
#48418=DIRECTION('',(0.,1.,0.));
#48419=DIRECTION('',(-0.838443593764828,0.,-0.544988385265888));
#48420=DIRECTION('center_axis',(0.,1.,0.));
#48421=DIRECTION('ref_axis',(1.,0.,0.));
#48422=DIRECTION('',(-0.492017200046991,0.,0.870585478202984));
#48423=DIRECTION('',(0.61395827519323,0.,0.789338480198295));
#48424=DIRECTION('center_axis',(0.,1.,0.));
#48425=DIRECTION('ref_axis',(1.,0.,0.));
#48426=DIRECTION('',(-0.977071912385473,0.,-0.212909553631103));
#48427=DIRECTION('center_axis',(-0.789338480198295,0.,0.61395827519323));
#48428=DIRECTION('ref_axis',(0.,1.,0.));
#48429=DIRECTION('',(-0.61395827519323,0.,-0.789338480198295));
#48430=DIRECTION('',(0.,1.,0.));
#48431=DIRECTION('',(0.,1.,0.));
#48432=DIRECTION('center_axis',(-0.870585478202985,0.,-0.492017200046991));
#48433=DIRECTION('ref_axis',(-0.492017200046991,0.,0.870585478202985));
#48434=DIRECTION('',(0.,1.,0.));
#48435=DIRECTION('',(0.492017200046991,0.,-0.870585478202984));
#48436=DIRECTION('center_axis',(0.212909553631103,0.,-0.977071912385473));
#48437=DIRECTION('ref_axis',(0.,-1.,0.));
#48438=DIRECTION('',(0.,1.,0.));
#48439=DIRECTION('',(0.977071912385473,0.,0.212909553631103));
#48440=DIRECTION('center_axis',(0.,-1.,0.));
#48441=DIRECTION('ref_axis',(0.,0.,-1.));
#48442=DIRECTION('center_axis',(0.,-1.,0.));
#48443=DIRECTION('ref_axis',(1.,0.,0.));
#48444=DIRECTION('center_axis',(0.,-1.,0.));
#48445=DIRECTION('ref_axis',(1.,0.,0.));
#48446=DIRECTION('',(0.,-1.,0.));
#48447=DIRECTION('center_axis',(0.,-1.,0.));
#48448=DIRECTION('ref_axis',(1.,0.,-1.8432640466762E-15));
#48449=DIRECTION('center_axis',(0.,-1.,0.));
#48450=DIRECTION('ref_axis',(0.,0.,-1.));
#48451=DIRECTION('',(-1.,0.,0.));
#48452=DIRECTION('center_axis',(0.,-1.,0.));
#48453=DIRECTION('ref_axis',(1.,0.,0.));
#48454=DIRECTION('',(0.,0.,-1.));
#48455=DIRECTION('center_axis',(0.,1.,0.));
#48456=DIRECTION('ref_axis',(1.,0.,0.));
#48457=DIRECTION('',(0.,0.,-1.));
#48458=DIRECTION('center_axis',(0.,-1.,0.));
#48459=DIRECTION('ref_axis',(1.,0.,0.));
#48460=DIRECTION('center_axis',(0.,1.,0.));
#48461=DIRECTION('ref_axis',(1.,0.,0.));
#48462=DIRECTION('',(-1.,0.,0.));
#48463=DIRECTION('center_axis',(0.,-1.,0.));
#48464=DIRECTION('ref_axis',(1.,0.,0.));
#48465=DIRECTION('center_axis',(0.,-1.,0.));
#48466=DIRECTION('ref_axis',(1.,0.,0.));
#48467=DIRECTION('',(0.,0.,-1.));
#48468=DIRECTION('center_axis',(0.,1.,0.));
#48469=DIRECTION('ref_axis',(1.,0.,0.));
#48470=DIRECTION('center_axis',(0.,1.,0.));
#48471=DIRECTION('ref_axis',(1.,0.,0.));
#48472=DIRECTION('center_axis',(0.,-1.,0.));
#48473=DIRECTION('ref_axis',(1.,0.,0.));
#48474=DIRECTION('center_axis',(0.,-1.,0.));
#48475=DIRECTION('ref_axis',(1.,0.,0.));
#48476=DIRECTION('center_axis',(0.,1.,0.));
#48477=DIRECTION('ref_axis',(1.,0.,0.));
#48478=DIRECTION('center_axis',(0.,1.,0.));
#48479=DIRECTION('ref_axis',(1.,0.,0.));
#48480=DIRECTION('center_axis',(0.,1.,0.));
#48481=DIRECTION('ref_axis',(1.,0.,0.));
#48482=DIRECTION('',(0.,0.,-1.));
#48483=DIRECTION('center_axis',(0.,1.,0.));
#48484=DIRECTION('ref_axis',(1.,0.,0.));
#48485=DIRECTION('center_axis',(0.,-1.,0.));
#48486=DIRECTION('ref_axis',(1.,0.,0.));
#48487=DIRECTION('',(-1.,0.,0.));
#48488=DIRECTION('center_axis',(0.,1.,0.));
#48489=DIRECTION('ref_axis',(1.,0.,0.));
#48490=DIRECTION('center_axis',(0.,-1.,0.));
#48491=DIRECTION('ref_axis',(1.,0.,0.));
#48492=DIRECTION('',(0.,0.,-1.));
#48493=DIRECTION('center_axis',(0.,1.,0.));
#48494=DIRECTION('ref_axis',(1.,0.,0.));
#48495=DIRECTION('',(0.,0.,-1.));
#48496=DIRECTION('center_axis',(0.,-1.,0.));
#48497=DIRECTION('ref_axis',(1.,0.,0.));
#48498=DIRECTION('',(-1.,0.,0.));
#48499=DIRECTION('center_axis',(6.12323399573677E-17,1.,0.));
#48500=DIRECTION('ref_axis',(1.,0.,0.));
#48501=DIRECTION('center_axis',(0.,0.,1.));
#48502=DIRECTION('ref_axis',(1.,0.,0.));
#48503=DIRECTION('center_axis',(0.,1.,0.));
#48504=DIRECTION('ref_axis',(1.,0.,0.));
#48505=DIRECTION('center_axis',(0.,1.,0.));
#48506=DIRECTION('ref_axis',(1.,0.,0.));
#48507=DIRECTION('',(-1.,0.,0.));
#48508=DIRECTION('center_axis',(0.,1.,0.));
#48509=DIRECTION('ref_axis',(1.,0.,0.));
#48510=DIRECTION('',(0.,0.,-1.));
#48511=DIRECTION('',(-1.,0.,0.));
#48512=DIRECTION('',(0.,0.,-1.));
#48513=DIRECTION('',(-1.,0.,0.));
#48514=DIRECTION('',(0.,0.,-1.));
#48515=DIRECTION('center_axis',(0.,1.,0.));
#48516=DIRECTION('ref_axis',(1.,0.,0.));
#48517=DIRECTION('',(-1.,0.,0.));
#48518=DIRECTION('center_axis',(0.,1.,0.));
#48519=DIRECTION('ref_axis',(1.,0.,0.));
#48520=DIRECTION('',(0.,0.,-1.));
#48521=DIRECTION('center_axis',(0.,1.,0.));
#48522=DIRECTION('ref_axis',(1.,0.,0.));
#48523=DIRECTION('center_axis',(0.,1.,0.));
#48524=DIRECTION('ref_axis',(1.,0.,0.));
#48525=DIRECTION('center_axis',(0.,1.,0.));
#48526=DIRECTION('ref_axis',(1.,0.,0.));
#48527=DIRECTION('center_axis',(-1.,0.,0.));
#48528=DIRECTION('ref_axis',(0.,0.,1.));
#48529=DIRECTION('',(0.,0.,1.));
#48530=DIRECTION('',(0.,-1.,0.));
#48531=DIRECTION('',(0.,-1.,0.));
#48532=DIRECTION('',(0.,0.,-1.));
#48533=DIRECTION('',(0.,-1.,0.));
#48534=DIRECTION('',(0.,-1.,0.));
#48535=DIRECTION('center_axis',(1.,0.,0.));
#48536=DIRECTION('ref_axis',(0.,0.707106781186548,-0.707106781186547));
#48537=DIRECTION('',(1.,0.,0.));
#48538=DIRECTION('center_axis',(1.,0.,0.));
#48539=DIRECTION('ref_axis',(0.,0.707106781186548,-0.707106781186547));
#48540=DIRECTION('center_axis',(1.,0.,0.));
#48541=DIRECTION('ref_axis',(0.,1.,0.));
#48542=DIRECTION('',(0.,1.,0.));
#48543=DIRECTION('',(0.,0.,1.));
#48544=DIRECTION('',(0.,1.,0.));
#48545=DIRECTION('center_axis',(1.,0.,0.));
#48546=DIRECTION('ref_axis',(0.,1.,0.));
#48547=DIRECTION('',(0.,-1.,0.));
#48548=DIRECTION('',(0.,0.,-1.));
#48549=DIRECTION('center_axis',(0.,-1.,0.));
#48550=DIRECTION('ref_axis',(0.,0.,-1.));
#48551=DIRECTION('',(-1.,0.,0.));
#48552=DIRECTION('center_axis',(0.,1.,0.));
#48553=DIRECTION('ref_axis',(1.,0.,0.));
#48554=DIRECTION('center_axis',(0.,0.,-1.));
#48555=DIRECTION('ref_axis',(0.,-1.,0.));
#48556=DIRECTION('',(0.,-1.,0.));
#48557=DIRECTION('',(1.,0.,0.));
#48558=DIRECTION('center_axis',(1.,0.,0.));
#48559=DIRECTION('ref_axis',(0.,0.,1.));
#48560=DIRECTION('',(-1.,0.,0.));
#48561=DIRECTION('center_axis',(0.,0.,1.));
#48562=DIRECTION('ref_axis',(1.,0.,0.));
#48563=DIRECTION('',(0.,-1.,0.));
#48564=DIRECTION('',(-1.,0.,0.));
#48565=DIRECTION('center_axis',(0.,1.,0.));
#48566=DIRECTION('ref_axis',(1.,0.,0.));
#48567=DIRECTION('center_axis',(0.,1.,0.));
#48568=DIRECTION('ref_axis',(1.,0.,0.));
#48569=DIRECTION('center_axis',(0.,-1.,0.));
#48570=DIRECTION('ref_axis',(0.,0.,-1.));
#48571=DIRECTION('center_axis',(0.,-1.,0.));
#48572=DIRECTION('ref_axis',(1.,0.,0.));
#48573=DIRECTION('',(0.,0.,1.));
#48574=DIRECTION('',(-1.,0.,0.));
#48575=DIRECTION('center_axis',(1.,0.,0.));
#48576=DIRECTION('ref_axis',(0.,1.,0.));
#48577=DIRECTION('',(0.,1.,0.));
#48578=DIRECTION('',(0.,0.,-1.));
#48579=DIRECTION('center_axis',(1.,0.,0.));
#48580=DIRECTION('ref_axis',(0.,1.,0.));
#48581=DIRECTION('',(0.,1.,0.));
#48582=DIRECTION('center_axis',(0.,0.,1.));
#48583=DIRECTION('ref_axis',(1.,0.,0.));
#48584=DIRECTION('',(0.,-1.,0.));
#48585=DIRECTION('',(1.,0.,0.));
#48586=DIRECTION('center_axis',(1.,0.,0.));
#48587=DIRECTION('ref_axis',(0.,0.707106781186548,0.707106781186547));
#48588=DIRECTION('',(-1.,0.,0.));
#48589=DIRECTION('center_axis',(0.,-1.,0.));
#48590=DIRECTION('ref_axis',(0.,0.,-1.));
#48591=DIRECTION('center_axis',(0.,1.,0.));
#48592=DIRECTION('ref_axis',(1.,0.,0.));
#48593=DIRECTION('center_axis',(1.,0.,0.));
#48594=DIRECTION('ref_axis',(0.,1.,0.));
#48595=DIRECTION('',(0.,1.,0.));
#48596=DIRECTION('',(0.,0.,1.));
#48597=DIRECTION('',(0.,1.,0.));
#48598=DIRECTION('center_axis',(1.,0.,0.));
#48599=DIRECTION('ref_axis',(0.,1.,0.));
#48600=DIRECTION('',(0.,0.,-1.));
#48601=DIRECTION('center_axis',(0.,-1.,0.));
#48602=DIRECTION('ref_axis',(0.,0.,-1.));
#48603=DIRECTION('center_axis',(0.,1.,0.));
#48604=DIRECTION('ref_axis',(1.,0.,0.));
#48605=DIRECTION('',(-1.,0.,0.));
#48606=DIRECTION('center_axis',(1.,0.,0.));
#48607=DIRECTION('ref_axis',(0.,0.707106781187215,0.70710678118588));
#48608=DIRECTION('',(1.,0.,0.));
#48609=DIRECTION('center_axis',(0.,0.,1.));
#48610=DIRECTION('ref_axis',(1.,0.,0.));
#48611=DIRECTION('',(-1.,0.,0.));
#48612=DIRECTION('',(0.,-1.,0.));
#48613=DIRECTION('center_axis',(0.,-1.,0.));
#48614=DIRECTION('ref_axis',(0.,0.,-1.));
#48615=DIRECTION('center_axis',(0.,-1.,0.));
#48616=DIRECTION('ref_axis',(1.,0.,0.));
#48617=DIRECTION('center_axis',(0.,1.,0.));
#48618=DIRECTION('ref_axis',(1.,0.,0.));
#48619=DIRECTION('center_axis',(0.,1.,0.));
#48620=DIRECTION('ref_axis',(1.,0.,0.));
#48621=DIRECTION('',(0.,0.,1.));
#48622=DIRECTION('',(-1.,0.,0.));
#48623=DIRECTION('center_axis',(1.,0.,0.));
#48624=DIRECTION('ref_axis',(0.,1.,0.));
#48625=DIRECTION('',(0.,1.,0.));
#48626=DIRECTION('',(0.,0.,-1.));
#48627=DIRECTION('',(0.,-1.,0.));
#48628=DIRECTION('center_axis',(1.,0.,0.));
#48629=DIRECTION('ref_axis',(0.,1.,0.));
#48630=DIRECTION('',(0.,1.,0.));
#48631=DIRECTION('center_axis',(0.,0.,1.));
#48632=DIRECTION('ref_axis',(1.,0.,0.));
#48633=DIRECTION('',(-1.,0.,0.));
#48634=DIRECTION('',(0.,-1.,0.));
#48635=DIRECTION('center_axis',(1.,0.,0.));
#48636=DIRECTION('ref_axis',(0.,0.,1.));
#48637=DIRECTION('',(1.,0.,0.));
#48638=DIRECTION('center_axis',(0.,0.,-1.));
#48639=DIRECTION('ref_axis',(0.,-1.,0.));
#48640=DIRECTION('',(0.,-1.,0.));
#48641=DIRECTION('',(-1.,0.,0.));
#48642=DIRECTION('center_axis',(0.,-1.,0.));
#48643=DIRECTION('ref_axis',(0.,0.,-1.));
#48644=DIRECTION('center_axis',(0.,1.,0.));
#48645=DIRECTION('ref_axis',(1.,0.,0.));
#48646=DIRECTION('center_axis',(0.,1.,0.));
#48647=DIRECTION('ref_axis',(1.,0.,0.));
#48648=DIRECTION('center_axis',(0.,-1.,0.));
#48649=DIRECTION('ref_axis',(1.,0.,0.));
#48650=DIRECTION('',(0.,0.,-1.));
#48651=DIRECTION('center_axis',(0.,1.,0.));
#48652=DIRECTION('ref_axis',(1.,0.,0.));
#48653=DIRECTION('center_axis',(0.,-1.,0.));
#48654=DIRECTION('ref_axis',(1.,0.,0.));
#48655=DIRECTION('',(0.,0.,-1.));
#48656=DIRECTION('center_axis',(0.,1.,0.));
#48657=DIRECTION('ref_axis',(0.,0.,1.));
#48658=DIRECTION('',(0.,-1.,0.));
#48659=DIRECTION('',(0.,1.,0.));
#48660=DIRECTION('center_axis',(0.,1.,0.));
#48661=DIRECTION('ref_axis',(0.,0.,1.));
#48662=DIRECTION('',(0.,-1.,0.));
#48663=DIRECTION('',(0.,1.,0.));
#48664=DIRECTION('center_axis',(0.,-1.,0.));
#48665=DIRECTION('ref_axis',(0.,0.,-1.));
#48666=DIRECTION('center_axis',(0.,1.,0.));
#48667=DIRECTION('ref_axis',(1.,0.,0.));
#48668=DIRECTION('center_axis',(0.,-1.,0.));
#48669=DIRECTION('ref_axis',(1.,0.,0.));
#48670=DIRECTION('',(-1.,0.,0.));
#48671=DIRECTION('center_axis',(0.,-1.,0.));
#48672=DIRECTION('ref_axis',(1.,0.,0.));
#48673=DIRECTION('center_axis',(-1.,0.,0.));
#48674=DIRECTION('ref_axis',(0.,0.,1.));
#48675=DIRECTION('',(0.,0.,-1.));
#48676=DIRECTION('center_axis',(-1.,0.,0.));
#48677=DIRECTION('ref_axis',(0.,0.,1.));
#48678=DIRECTION('',(0.,0.,-1.));
#48679=DIRECTION('center_axis',(0.,-1.,0.));
#48680=DIRECTION('ref_axis',(3.06161699786735E-16,0.,1.));
#48681=DIRECTION('center_axis',(0.,1.,0.));
#48682=DIRECTION('ref_axis',(1.,0.,0.));
#48683=DIRECTION('',(0.,1.,0.));
#48684=DIRECTION('',(0.,-1.,0.));
#48685=DIRECTION('center_axis',(0.,-1.,0.));
#48686=DIRECTION('ref_axis',(-0.707106781186548,0.,-0.707106781186548));
#48687=DIRECTION('center_axis',(0.,-1.,0.));
#48688=DIRECTION('ref_axis',(1.,0.,0.));
#48689=DIRECTION('',(0.,-1.,0.));
#48690=DIRECTION('center_axis',(0.,0.,1.));
#48691=DIRECTION('ref_axis',(1.,0.,0.));
#48692=DIRECTION('',(0.,-1.,0.));
#48693=DIRECTION('',(-1.,0.,0.));
#48694=DIRECTION('center_axis',(0.,-1.,0.));
#48695=DIRECTION('ref_axis',(0.707106781186548,0.,-0.707106781186548));
#48696=DIRECTION('center_axis',(0.,-1.,0.));
#48697=DIRECTION('ref_axis',(1.,0.,0.));
#48698=DIRECTION('center_axis',(1.,0.,0.));
#48699=DIRECTION('ref_axis',(0.,0.707106781186548,-0.707106781186547));
#48700=DIRECTION('center_axis',(-1.,0.,0.));
#48701=DIRECTION('ref_axis',(0.,0.707106781186548,-0.707106781186547));
#48702=DIRECTION('',(1.,0.,0.));
#48703=DIRECTION('center_axis',(0.,-1.,0.));
#48704=DIRECTION('ref_axis',(0.,0.,-1.));
#48705=DIRECTION('center_axis',(0.,-1.,0.));
#48706=DIRECTION('ref_axis',(1.,0.,0.));
#48707=DIRECTION('',(1.,0.,0.));
#48708=DIRECTION('',(0.,0.,-1.));
#48709=DIRECTION('center_axis',(0.,0.,-1.));
#48710=DIRECTION('ref_axis',(0.,-1.,0.));
#48711=DIRECTION('',(0.,-1.,0.));
#48712=DIRECTION('',(-1.,0.,0.));
#48713=DIRECTION('',(0.,-1.,0.));
#48714=DIRECTION('center_axis',(1.,0.,0.));
#48715=DIRECTION('ref_axis',(0.,0.,1.));
#48716=DIRECTION('',(1.,0.,0.));
#48717=DIRECTION('center_axis',(1.,0.,0.));
#48718=DIRECTION('ref_axis',(0.,1.,0.));
#48719=DIRECTION('center_axis',(0.,0.,1.));
#48720=DIRECTION('ref_axis',(1.,0.,0.));
#48721=DIRECTION('',(-1.,0.,0.));
#48722=DIRECTION('',(0.,1.,0.));
#48723=DIRECTION('',(0.,-1.,0.));
#48724=DIRECTION('center_axis',(0.,0.,1.));
#48725=DIRECTION('ref_axis',(1.,0.,0.));
#48726=DIRECTION('',(0.,-1.,0.));
#48727=DIRECTION('',(1.,0.,0.));
#48728=DIRECTION('',(0.,1.,0.));
#48729=DIRECTION('',(-1.,0.,0.));
#48730=DIRECTION('center_axis',(1.,0.,0.));
#48731=DIRECTION('ref_axis',(0.,0.,1.));
#48732=DIRECTION('',(-1.,0.,0.));
#48733=DIRECTION('center_axis',(1.,0.,0.));
#48734=DIRECTION('ref_axis',(0.,1.,0.));
#48735=DIRECTION('center_axis',(0.,0.,-1.));
#48736=DIRECTION('ref_axis',(0.,-1.,0.));
#48737=DIRECTION('',(0.,-1.,0.));
#48738=DIRECTION('',(0.,-1.,0.));
#48739=DIRECTION('',(1.,0.,0.));
#48740=DIRECTION('center_axis',(0.,-1.,0.));
#48741=DIRECTION('ref_axis',(0.,0.,-1.));
#48742=DIRECTION('center_axis',(0.,-1.,0.));
#48743=DIRECTION('ref_axis',(1.,0.,0.));
#48744=DIRECTION('',(0.,0.,-1.));
#48745=DIRECTION('center_axis',(0.,-1.,0.));
#48746=DIRECTION('ref_axis',(0.,0.,-1.));
#48747=DIRECTION('',(0.,0.,-1.));
#48748=DIRECTION('center_axis',(0.,-1.,0.));
#48749=DIRECTION('ref_axis',(1.,0.,0.));
#48750=DIRECTION('',(1.,0.,0.));
#48751=DIRECTION('center_axis',(1.,0.,0.));
#48752=DIRECTION('ref_axis',(0.,0.707106781187215,0.70710678118588));
#48753=DIRECTION('',(-1.,0.,0.));
#48754=DIRECTION('center_axis',(1.,0.,0.));
#48755=DIRECTION('ref_axis',(0.,1.,0.));
#48756=DIRECTION('center_axis',(0.,0.,1.));
#48757=DIRECTION('ref_axis',(1.,0.,0.));
#48758=DIRECTION('',(0.,-1.,0.));
#48759=DIRECTION('',(-1.,0.,0.));
#48760=DIRECTION('',(0.,1.,0.));
#48761=DIRECTION('center_axis',(0.,-1.,0.));
#48762=DIRECTION('ref_axis',(0.,0.,-1.));
#48763=DIRECTION('',(0.,0.,-1.));
#48764=DIRECTION('',(1.,0.,0.));
#48765=DIRECTION('center_axis',(0.,-1.,0.));
#48766=DIRECTION('ref_axis',(1.,0.,0.));
#48767=DIRECTION('center_axis',(1.,0.,0.));
#48768=DIRECTION('ref_axis',(0.,0.707106781186548,0.707106781186547));
#48769=DIRECTION('',(-1.,0.,0.));
#48770=DIRECTION('center_axis',(1.,0.,0.));
#48771=DIRECTION('ref_axis',(0.,1.,0.));
#48772=DIRECTION('center_axis',(0.,0.,1.));
#48773=DIRECTION('ref_axis',(1.,0.,0.));
#48774=DIRECTION('',(0.,1.,0.));
#48775=DIRECTION('',(-1.,0.,0.));
#48776=DIRECTION('',(0.,-1.,0.));
#48777=DIRECTION('center_axis',(0.,0.,-1.));
#48778=DIRECTION('ref_axis',(1.,0.,0.));
#48779=DIRECTION('center_axis',(-6.12323399574E-17,0.,1.));
#48780=DIRECTION('ref_axis',(1.,0.,6.12323399574E-17));
#48781=DIRECTION('center_axis',(2.96059473233E-15,0.,1.));
#48782=DIRECTION('ref_axis',(1.,0.,-2.96059473233E-15));
#48783=DIRECTION('',(0.,0.,1.));
#48784=DIRECTION('center_axis',(0.,1.,0.));
#48785=DIRECTION('ref_axis',(1.,0.,0.));
#48786=DIRECTION('',(-1.,0.,0.));
#48787=DIRECTION('center_axis',(0.,-1.,0.));
#48788=DIRECTION('ref_axis',(1.,0.,0.));
#48789=DIRECTION('center_axis',(0.,1.,0.));
#48790=DIRECTION('ref_axis',(1.,0.,0.));
#48791=DIRECTION('',(0.,0.,-1.));
#48792=DIRECTION('center_axis',(0.,1.,0.));
#48793=DIRECTION('ref_axis',(1.,0.,0.));
#48794=DIRECTION('center_axis',(0.,-1.,0.));
#48795=DIRECTION('ref_axis',(1.,0.,0.));
#48796=DIRECTION('center_axis',(0.,1.,0.));
#48797=DIRECTION('ref_axis',(1.,0.,0.));
#48798=DIRECTION('center_axis',(0.,1.,0.));
#48799=DIRECTION('ref_axis',(1.,0.,0.));
#48800=DIRECTION('center_axis',(0.,-1.,0.));
#48801=DIRECTION('ref_axis',(1.,0.,0.));
#48802=DIRECTION('center_axis',(0.,1.,0.));
#48803=DIRECTION('ref_axis',(1.,0.,0.));
#48804=DIRECTION('',(0.,0.,-1.));
#48805=DIRECTION('center_axis',(0.,1.,0.));
#48806=DIRECTION('ref_axis',(1.,0.,0.));
#48807=DIRECTION('center_axis',(0.,-1.,0.));
#48808=DIRECTION('ref_axis',(1.,0.,0.));
#48809=DIRECTION('center_axis',(0.,1.,0.));
#48810=DIRECTION('ref_axis',(1.,0.,0.));
#48811=DIRECTION('',(0.,0.,1.));
#48812=DIRECTION('center_axis',(0.,1.,0.));
#48813=DIRECTION('ref_axis',(1.,0.,0.));
#48814=DIRECTION('center_axis',(0.,-1.,0.));
#48815=DIRECTION('ref_axis',(1.,0.,0.));
#48816=DIRECTION('center_axis',(0.,1.,0.));
#48817=DIRECTION('ref_axis',(1.,0.,0.));
#48818=DIRECTION('center_axis',(0.,1.,0.));
#48819=DIRECTION('ref_axis',(1.,0.,0.));
#48820=DIRECTION('center_axis',(0.,-1.,0.));
#48821=DIRECTION('ref_axis',(1.,0.,0.));
#48822=DIRECTION('center_axis',(0.,1.,0.));
#48823=DIRECTION('ref_axis',(1.,0.,0.));
#48824=DIRECTION('',(0.,0.,-1.));
#48825=DIRECTION('center_axis',(0.,1.,0.));
#48826=DIRECTION('ref_axis',(1.,0.,0.));
#48827=DIRECTION('center_axis',(0.,-1.,0.));
#48828=DIRECTION('ref_axis',(1.,0.,0.));
#48829=DIRECTION('',(-1.,0.,0.));
#48830=DIRECTION('center_axis',(0.,-1.,0.));
#48831=DIRECTION('ref_axis',(1.,0.,0.));
#48832=DIRECTION('center_axis',(0.,1.,0.));
#48833=DIRECTION('ref_axis',(1.,0.,0.));
#48834=DIRECTION('center_axis',(0.,1.,0.));
#48835=DIRECTION('ref_axis',(1.,0.,0.));
#48836=DIRECTION('',(1.,0.,0.));
#48837=DIRECTION('center_axis',(0.,1.,0.));
#48838=DIRECTION('ref_axis',(1.,0.,0.));
#48839=DIRECTION('',(0.,0.,-1.));
#48840=DIRECTION('center_axis',(0.,1.,0.));
#48841=DIRECTION('ref_axis',(1.,0.,0.));
#48842=DIRECTION('center_axis',(0.,-1.,0.));
#48843=DIRECTION('ref_axis',(-0.873189157202533,0.,0.487381468404298));
#48844=DIRECTION('',(0.,-1.,0.));
#48845=DIRECTION('',(0.,1.,0.));
#48846=DIRECTION('center_axis',(0.,-1.,0.));
#48847=DIRECTION('ref_axis',(1.,0.,0.));
#48848=DIRECTION('center_axis',(0.,0.,-1.));
#48849=DIRECTION('ref_axis',(0.,-1.,0.));
#48850=DIRECTION('',(0.,-1.,0.));
#48851=DIRECTION('',(-1.,0.,0.));
#48852=DIRECTION('center_axis',(0.,-1.,0.));
#48853=DIRECTION('ref_axis',(3.06161699786735E-16,0.,1.));
#48854=DIRECTION('center_axis',(0.,-1.,0.));
#48855=DIRECTION('ref_axis',(1.,0.,0.));
#48856=DIRECTION('',(0.,-1.,0.));
#48857=DIRECTION('center_axis',(0.,0.,-1.));
#48858=DIRECTION('ref_axis',(0.,-1.,0.));
#48859=DIRECTION('',(0.,1.,0.));
#48860=DIRECTION('',(-1.,0.,0.));
#48861=DIRECTION('center_axis',(0.,-1.,0.));
#48862=DIRECTION('ref_axis',(0.543088776464994,0.,-0.839675282997991));
#48863=DIRECTION('',(0.,-1.,0.));
#48864=DIRECTION('center_axis',(0.,-1.,0.));
#48865=DIRECTION('ref_axis',(1.,0.,0.));
#48866=DIRECTION('center_axis',(0.,1.,0.));
#48867=DIRECTION('ref_axis',(-1.,0.,0.));
#48868=DIRECTION('',(0.,-1.,0.));
#48869=DIRECTION('center_axis',(0.,-1.,0.));
#48870=DIRECTION('ref_axis',(1.,0.,0.));
#48871=DIRECTION('center_axis',(1.,0.,0.));
#48872=DIRECTION('ref_axis',(0.,1.,0.));
#48873=DIRECTION('',(0.,1.,0.));
#48874=DIRECTION('',(0.,0.,1.));
#48875=DIRECTION('center_axis',(0.,-1.,0.));
#48876=DIRECTION('ref_axis',(0.418360127903027,0.,-0.90828123584106));
#48877=DIRECTION('center_axis',(0.,-1.,0.));
#48878=DIRECTION('ref_axis',(1.,0.,0.));
#48879=DIRECTION('',(0.,1.,0.));
#48880=DIRECTION('center_axis',(0.,-1.,0.));
#48881=DIRECTION('ref_axis',(-0.429581475917968,0.,-0.903028103409933));
#48882=DIRECTION('center_axis',(0.,-1.,0.));
#48883=DIRECTION('ref_axis',(1.,0.,0.));
#48884=DIRECTION('',(0.,1.,0.));
#48885=DIRECTION('center_axis',(0.,1.,0.));
#48886=DIRECTION('ref_axis',(0.344636603387807,0.,-0.938736177850473));
#48887=DIRECTION('center_axis',(0.,-1.,0.));
#48888=DIRECTION('ref_axis',(1.,0.,0.));
#48889=DIRECTION('',(0.,-1.,0.));
#48890=DIRECTION('center_axis',(0.,1.,0.));
#48891=DIRECTION('ref_axis',(-0.307788100148132,0.,0.951454930833407));
#48892=DIRECTION('',(0.,-1.,0.));
#48893=DIRECTION('center_axis',(0.,-1.,0.));
#48894=DIRECTION('ref_axis',(1.,0.,0.));
#48895=DIRECTION('center_axis',(0.,-1.,0.));
#48896=DIRECTION('ref_axis',(-0.329929783129,0.,-0.944005475728002));
#48897=DIRECTION('',(0.,-1.,0.));
#48898=DIRECTION('center_axis',(0.,-1.,0.));
#48899=DIRECTION('ref_axis',(1.,0.,0.));
#48900=DIRECTION('center_axis',(0.,1.,0.));
#48901=DIRECTION('ref_axis',(-1.,0.,0.));
#48902=DIRECTION('',(0.,-1.,0.));
#48903=DIRECTION('center_axis',(0.,-1.,0.));
#48904=DIRECTION('ref_axis',(1.,0.,0.));
#48905=DIRECTION('center_axis',(1.,0.,0.));
#48906=DIRECTION('ref_axis',(0.,1.,0.));
#48907=DIRECTION('',(0.,0.,1.));
#48908=DIRECTION('',(0.,1.,0.));
#48909=DIRECTION('center_axis',(0.,-1.,0.));
#48910=DIRECTION('ref_axis',(0.186470178118022,0.,-0.982460621436113));
#48911=DIRECTION('center_axis',(0.,-1.,0.));
#48912=DIRECTION('ref_axis',(1.,0.,0.));
#48913=DIRECTION('',(0.,1.,0.));
#48914=DIRECTION('center_axis',(0.,-1.,0.));
#48915=DIRECTION('ref_axis',(-0.429581475917968,0.,-0.903028103409933));
#48916=DIRECTION('',(0.,1.,0.));
#48917=DIRECTION('center_axis',(0.,-1.,0.));
#48918=DIRECTION('ref_axis',(1.,0.,0.));
#48919=DIRECTION('center_axis',(0.,1.,0.));
#48920=DIRECTION('ref_axis',(-0.186470178118022,0.,-0.982460621436113));
#48921=DIRECTION('center_axis',(0.,-1.,0.));
#48922=DIRECTION('ref_axis',(1.,0.,0.));
#48923=DIRECTION('',(0.,1.,0.));
#48924=DIRECTION('center_axis',(1.,0.,0.));
#48925=DIRECTION('ref_axis',(0.,1.,0.));
#48926=DIRECTION('',(0.,-1.,0.));
#48927=DIRECTION('',(0.,0.,-1.));
#48928=DIRECTION('center_axis',(0.,-1.,0.));
#48929=DIRECTION('ref_axis',(1.,0.,1.15648231731787E-14));
#48930=DIRECTION('',(0.,-1.,0.));
#48931=DIRECTION('center_axis',(0.,-1.,0.));
#48932=DIRECTION('ref_axis',(1.,0.,0.));
#48933=DIRECTION('center_axis',(0.,-1.,0.));
#48934=DIRECTION('ref_axis',(-0.329929783129,0.,-0.944005475728002));
#48935=DIRECTION('',(0.,-1.,0.));
#48936=DIRECTION('center_axis',(0.,-1.,0.));
#48937=DIRECTION('ref_axis',(1.,0.,0.));
#48938=DIRECTION('center_axis',(0.,1.,0.));
#48939=DIRECTION('ref_axis',(-1.,0.,0.));
#48940=DIRECTION('',(0.,1.,0.));
#48941=DIRECTION('center_axis',(0.,-1.,0.));
#48942=DIRECTION('ref_axis',(1.,0.,0.));
#48943=DIRECTION('center_axis',(0.,1.,0.));
#48944=DIRECTION('ref_axis',(0.902179063668487,0.,-0.43136172416923));
#48945=DIRECTION('center_axis',(0.,-1.,0.));
#48946=DIRECTION('ref_axis',(1.,0.,0.));
#48947=DIRECTION('',(0.,1.,0.));
#48948=DIRECTION('center_axis',(0.,-1.,0.));
#48949=DIRECTION('ref_axis',(-0.429581475917968,0.,-0.903028103409933));
#48950=DIRECTION('',(0.,1.,0.));
#48951=DIRECTION('center_axis',(0.,-1.,0.));
#48952=DIRECTION('ref_axis',(1.,0.,0.));
#48953=DIRECTION('center_axis',(0.,1.,0.));
#48954=DIRECTION('ref_axis',(-0.418360127903027,0.,-0.90828123584106));
#48955=DIRECTION('center_axis',(0.,-1.,0.));
#48956=DIRECTION('ref_axis',(1.,0.,0.));
#48957=DIRECTION('',(0.,1.,0.));
#48958=DIRECTION('center_axis',(1.,0.,0.));
#48959=DIRECTION('ref_axis',(0.,1.,0.));
#48960=DIRECTION('',(0.,-1.,0.));
#48961=DIRECTION('',(0.,0.,-1.));
#48962=DIRECTION('center_axis',(0.,-1.,0.));
#48963=DIRECTION('ref_axis',(1.,0.,5.78241158658936E-15));
#48964=DIRECTION('center_axis',(0.,-1.,0.));
#48965=DIRECTION('ref_axis',(1.,0.,0.));
#48966=DIRECTION('center_axis',(0.,-1.,0.));
#48967=DIRECTION('ref_axis',(0.,0.,-1.));
#48968=DIRECTION('center_axis',(0.,-1.,0.));
#48969=DIRECTION('ref_axis',(1.,0.,0.));
#48970=DIRECTION('',(0.,0.,1.));
#48971=DIRECTION('center_axis',(1.,0.,0.));
#48972=DIRECTION('ref_axis',(0.,1.,0.));
#48973=DIRECTION('',(0.,1.,0.));
#48974=DIRECTION('center_axis',(1.,0.,0.));
#48975=DIRECTION('ref_axis',(0.,1.,0.));
#48976=DIRECTION('',(0.,1.,0.));
#48977=DIRECTION('',(0.,0.,1.));
#48978=DIRECTION('center_axis',(0.,1.,0.));
#48979=DIRECTION('ref_axis',(1.,0.,0.));
#48980=DIRECTION('center_axis',(0.,1.,0.));
#48981=DIRECTION('ref_axis',(1.,0.,0.));
#48982=DIRECTION('center_axis',(0.,1.,0.));
#48983=DIRECTION('ref_axis',(1.,0.,0.));
#48984=DIRECTION('center_axis',(0.,1.,0.));
#48985=DIRECTION('ref_axis',(1.,0.,0.));
#48986=DIRECTION('',(0.,0.,1.));
#48987=DIRECTION('center_axis',(1.,0.,0.));
#48988=DIRECTION('ref_axis',(0.,1.,0.));
#48989=DIRECTION('',(0.,1.,0.));
#48990=DIRECTION('center_axis',(0.,1.,0.));
#48991=DIRECTION('ref_axis',(1.07187543957E-15,0.,-1.));
#48992=DIRECTION('',(0.,-1.,0.));
#48993=DIRECTION('center_axis',(0.,-1.,0.));
#48994=DIRECTION('ref_axis',(1.,0.,0.));
#48995=DIRECTION('center_axis',(0.,-1.,0.));
#48996=DIRECTION('ref_axis',(1.,0.,0.));
#48997=DIRECTION('',(0.,1.,0.));
#48998=DIRECTION('center_axis',(1.,0.,0.));
#48999=DIRECTION('ref_axis',(0.,1.,0.));
#49000=DIRECTION('',(0.,0.,1.));
#49001=DIRECTION('center_axis',(0.,-1.,0.));
#49002=DIRECTION('ref_axis',(0.,0.,-1.));
#49003=DIRECTION('center_axis',(0.,1.,0.));
#49004=DIRECTION('ref_axis',(-1.,0.,0.));
#49005=DIRECTION('center_axis',(0.,1.,0.));
#49006=DIRECTION('ref_axis',(1.,0.,0.));
#49007=DIRECTION('center_axis',(1.,0.,0.));
#49008=DIRECTION('ref_axis',(0.,-1.,0.));
#49009=DIRECTION('center_axis',(0.,-1.,0.));
#49010=DIRECTION('ref_axis',(0.,0.,1.));
#49011=DIRECTION('',(0.,-1.,0.));
#49012=DIRECTION('center_axis',(-1.,0.,0.));
#49013=DIRECTION('ref_axis',(0.,0.,-1.));
#49014=DIRECTION('',(1.,0.,0.));
#49015=DIRECTION('center_axis',(1.,0.,0.));
#49016=DIRECTION('ref_axis',(0.,-1.,0.));
#49017=DIRECTION('center_axis',(0.,0.,1.));
#49018=DIRECTION('ref_axis',(1.,0.,0.));
#49019=DIRECTION('',(0.,-1.,0.));
#49020=DIRECTION('center_axis',(0.,1.,0.));
#49021=DIRECTION('ref_axis',(0.,0.,1.));
#49022=DIRECTION('center_axis',(0.,1.,0.));
#49023=DIRECTION('ref_axis',(1.,0.,0.));
#49024=DIRECTION('center_axis',(0.,0.,-1.));
#49025=DIRECTION('ref_axis',(1.,0.,0.));
#49026=DIRECTION('center_axis',(0.,-1.,0.));
#49027=DIRECTION('ref_axis',(1.,0.,0.));
#49028=DIRECTION('',(0.,-1.,0.));
#49029=DIRECTION('center_axis',(0.,0.,-1.));
#49030=DIRECTION('ref_axis',(0.,-1.,0.));
#49031=DIRECTION('',(0.,0.,-1.));
#49032=DIRECTION('center_axis',(-2.96059473233E-15,0.,-1.));
#49033=DIRECTION('ref_axis',(1.,0.,-2.96059473233E-15));
#49034=DIRECTION('center_axis',(-1.,0.,0.));
#49035=DIRECTION('ref_axis',(0.,0.,1.));
#49036=DIRECTION('',(0.,-1.,0.));
#49037=DIRECTION('center_axis',(-0.281178364446097,0.957593555167328,-0.0628753566146216));
#49038=DIRECTION('ref_axis',(0.959655525367003,0.280574208691291,-0.0184224333310672));
#49039=DIRECTION('center_axis',(-0.347084583568743,0.937833829550263,-7.75916811511616E-9));
#49040=DIRECTION('ref_axis',(-0.000199174768141593,-7.37046693238533E-5,
0.999999977448517));
#49041=DIRECTION('center_axis',(0.402792847081471,-0.209438030836135,0.891007089522572));
#49042=DIRECTION('ref_axis',(0.142300775827966,-0.947302276471775,-0.286999801724934));
#49043=DIRECTION('center_axis',(-0.975898622063701,0.,-0.218224378688931));
#49044=DIRECTION('ref_axis',(0.218224378688931,0.,-0.975898622063701));
#49045=DIRECTION('center_axis',(0.,1.,0.));
#49046=DIRECTION('ref_axis',(1.,0.,0.));
#49047=DIRECTION('center_axis',(0.,1.,0.));
#49048=DIRECTION('ref_axis',(1.,0.,0.));
#49049=DIRECTION('center_axis',(0.,-1.,0.));
#49050=DIRECTION('ref_axis',(0.,0.,-1.));
#49051=DIRECTION('',(0.,-1.,0.));
#49052=DIRECTION('center_axis',(0.,0.,1.));
#49053=DIRECTION('ref_axis',(1.,1.04089100950122E-14,0.));
#49054=DIRECTION('center_axis',(0.,0.,1.));
#49055=DIRECTION('ref_axis',(1.,0.,0.));
#49056=DIRECTION('center_axis',(-0.347083730899991,-0.937834145110104,3.18494860620805E-6));
#49057=DIRECTION('ref_axis',(0.000200278976134303,-7.07253260845549E-5,
0.99999997744313));
#49058=DIRECTION('center_axis',(0.,0.,1.));
#49059=DIRECTION('ref_axis',(1.,0.,0.));
#49060=DIRECTION('',(0.,-1.,0.));
#49061=DIRECTION('center_axis',(-0.281178364446097,-0.957593555167328,0.0628753566146216));
#49062=DIRECTION('ref_axis',(0.959655525367003,-0.280574208691291,0.0184224333310672));
#49063=DIRECTION('center_axis',(-0.359750052411863,-0.876095983477336,0.320991787316344));
#49064=DIRECTION('ref_axis',(-0.230372498903045,0.416775382555072,0.879333152022167));
#49065=DIRECTION('center_axis',(0.975898622063701,0.,-0.218224378688931));
#49066=DIRECTION('ref_axis',(0.218224378688931,0.,0.975898622063701));
#49067=DIRECTION('center_axis',(0.,1.,0.));
#49068=DIRECTION('ref_axis',(0.,0.,-1.));
#49069=DIRECTION('center_axis',(0.,1.,0.));
#49070=DIRECTION('ref_axis',(1.,0.,0.));
#49071=DIRECTION('center_axis',(0.,-1.,0.));
#49072=DIRECTION('ref_axis',(-1.,0.,0.));
#49073=DIRECTION('center_axis',(0.,-1.,0.));
#49074=DIRECTION('ref_axis',(0.,0.,-1.));
#49075=DIRECTION('center_axis',(0.,0.,-1.));
#49076=DIRECTION('ref_axis',(0.,-1.,0.));
#49077=DIRECTION('',(1.,0.,0.));
#49078=DIRECTION('',(0.,-1.,0.));
#49079=DIRECTION('center_axis',(1.,0.,0.));
#49080=DIRECTION('ref_axis',(0.,1.,0.));
#49081=DIRECTION('',(0.,0.,-1.));
#49082=DIRECTION('',(0.,-1.,0.));
#49083=DIRECTION('center_axis',(0.,1.,0.));
#49084=DIRECTION('ref_axis',(1.,0.,0.));
#49085=DIRECTION('',(1.,0.,0.));
#49086=DIRECTION('center_axis',(0.,0.,-1.));
#49087=DIRECTION('ref_axis',(0.,-1.,0.));
#97330=CARTESIAN_POINT('',(0.,0.,0.));
#97331=CARTESIAN_POINT('Origin',(1.33226762955E-14,-19.0742356128,-4.4019615652));
#97332=CARTESIAN_POINT('',(-4.33093462721,-19.3742356128,-6.08690818754));
#97333=CARTESIAN_POINT('',(-3.63173186089,-19.3742356128,-7.3013690143));
#97334=CARTESIAN_POINT('Origin',(8.59173843182E-14,-19.3742356128,-4.4019615652));
#97335=CARTESIAN_POINT('',(3.63173186095,-19.3742356128,-7.3013690143));
#97336=CARTESIAN_POINT('Origin',(1.33226762955E-14,-19.3742356128,-4.4019615652));
#97337=CARTESIAN_POINT('',(4.33093462721,-19.3742356128,-6.08690818754));
#97338=CARTESIAN_POINT('Origin',(7.66166644017E-14,-19.3742356128,-4.4019615652));
#97339=CARTESIAN_POINT('',(4.05968610969081,-19.146953327667,-5.98137915983575));
#97340=CARTESIAN_POINT('Origin',(4.33093462721,-19.0742356128,-6.08690818754));
#97341=CARTESIAN_POINT('',(-4.0596861374133,-19.1469533408308,-5.98137909746699));
#97342=CARTESIAN_POINT('Origin',(1.33226762955E-14,-19.146953353,-4.4019615652));
#97343=CARTESIAN_POINT('Origin',(-4.33093462721,-19.0742356128,-6.08690818754));
#97344=CARTESIAN_POINT('Origin',(0.,-3.07423561284,0.473661560394));
#97345=CARTESIAN_POINT('',(5.42382962926,-3.07423561284,7.46684196367));
#97346=CARTESIAN_POINT('',(6.97990993744,-3.07423561284,5.91455829396));
#97347=CARTESIAN_POINT('Origin',(0.,-3.07423561284,0.473661560394));
#97348=CARTESIAN_POINT('',(5.65920103905,-3.07423561284,5.05609743232));
#97349=CARTESIAN_POINT('',(6.31955548824,-3.07423561284,5.48532786314));
#97350=CARTESIAN_POINT('',(4.5,-3.07423561284,6.1986309857));
#97351=CARTESIAN_POINT('Origin',(0.,-3.07423561284,0.473661560394));
#97352=CARTESIAN_POINT('',(4.5,-3.07423561284,6.27570807841));
#97353=CARTESIAN_POINT('',(4.5,-3.07423561284,6.23716953205));
#97354=CARTESIAN_POINT('',(4.96191481463,-3.07423561284,6.87127502104));
#97355=CARTESIAN_POINT('Origin',(5.42382962926,-4.67423561284,7.46684196367));
#97356=CARTESIAN_POINT('',(4.5,-4.67423561284,6.27570807841));
#97357=CARTESIAN_POINT('',(4.5,-3.87423561284,6.27570807841));
#97358=CARTESIAN_POINT('',(5.42382962926,-4.67423561284,7.46684196367));
#97359=CARTESIAN_POINT('',(4.96191481463,-4.67423561284,6.87127502104));
#97360=CARTESIAN_POINT('',(5.42382962926,-12.0242356128,7.46684196367));
#97361=CARTESIAN_POINT('Origin',(4.5,-4.67423561284,6.27570807841));
#97362=CARTESIAN_POINT('',(4.5,-4.67423561284,6.1986309857));
#97363=CARTESIAN_POINT('',(4.5,-3.87423561284,6.1986309857));
#97364=CARTESIAN_POINT('',(4.5,-4.67423561284,6.23716953205));
#97365=CARTESIAN_POINT('Origin',(0.,-3.87423561284,0.473661560394));
#97366=CARTESIAN_POINT('',(5.65920103905,-4.67423561284,5.05609743232));
#97367=CARTESIAN_POINT('',(5.65920103905,-3.87423561284,5.05609743232));
#97368=CARTESIAN_POINT('Origin',(0.,-4.67423561284,0.473661560394));
#97369=CARTESIAN_POINT('Origin',(5.65920103905,-4.67423561284,5.05609743232));
#97370=CARTESIAN_POINT('',(6.97990993744,-4.67423561284,5.91455829396));
#97371=CARTESIAN_POINT('',(6.97990993744,-12.0242356128,5.91455829396));
#97372=CARTESIAN_POINT('',(6.31955548824,-4.67423561284,5.48532786314));
#97373=CARTESIAN_POINT('Origin',(0.,-1.97423561284,0.473661560394));
#97374=CARTESIAN_POINT('',(-4.68330338854,-1.97423561284,-4.73359921144));
#97375=CARTESIAN_POINT('',(-6.87681426213,-1.97423561284,-0.852355399956));
#97376=CARTESIAN_POINT('',(-5.78005882534,-1.97423561284,-2.7929773057));
#97377=CARTESIAN_POINT('',(-5.81927285325,-1.97423561284,-6.19406394831));
#97378=CARTESIAN_POINT('',(-5.2512881209,-1.97423561284,-5.46383157987));
#97379=CARTESIAN_POINT('',(-8.68139919901,-1.97423561284,-1.24558477082));
#97380=CARTESIAN_POINT('Origin',(0.,-1.97423561284,0.473661560394));
#97381=CARTESIAN_POINT('',(-7.77910673057,-1.97423561284,-1.04897008539));
#97382=CARTESIAN_POINT('Origin',(-5.81927285325,-4.67423561284,-6.19406394831));
#97383=CARTESIAN_POINT('',(-4.68330338854,-4.67423561284,-4.73359921144));
#97384=CARTESIAN_POINT('',(-5.81927285325,-4.67423561284,-6.19406394831));
#97385=CARTESIAN_POINT('',(-5.2512881209,-4.67423561284,-5.46383157987));
#97386=CARTESIAN_POINT('',(-5.81927285325,-12.0242356128,-6.19406394831));
#97387=CARTESIAN_POINT('',(-4.68330338854,-3.32423561284,-4.73359921144));
#97388=CARTESIAN_POINT('Origin',(-4.68330338854,-4.67423561284,-4.73359921144));
#97389=CARTESIAN_POINT('',(-6.87681426213,-4.67423561284,-0.852355399956));
#97390=CARTESIAN_POINT('',(-6.87681426213,-3.32423561284,-0.852355399956));
#97391=CARTESIAN_POINT('',(-5.78005882534,-4.67423561284,-2.7929773057));
#97392=CARTESIAN_POINT('Origin',(-6.87681426213,-4.67423561284,-0.852355399956));
#97393=CARTESIAN_POINT('',(-8.68139919901,-4.67423561284,-1.24558477082));
#97394=CARTESIAN_POINT('',(-8.68139919901,-12.0242356128,-1.24558477082));
#97395=CARTESIAN_POINT('',(-7.77910673057,-4.67423561284,-1.04897008539));
#97396=CARTESIAN_POINT('Origin',(0.,-18.3742356128,0.473661560394));
#97397=CARTESIAN_POINT('',(-1.2046272227,-18.3742356128,-11.8721618652));
#97398=CARTESIAN_POINT('Origin',(0.,-18.3742356128,-11.8721618652));
#97399=CARTESIAN_POINT('Origin',(0.,-18.8742356128,-11.8721618652));
#97400=CARTESIAN_POINT('',(-1.2046272227,-19.3742356128,-11.8721618652));
#97401=CARTESIAN_POINT('',(-1.2046272227,-18.8742356128,-11.8721618652));
#97402=CARTESIAN_POINT('Origin',(-4.16333634234434E-16,-19.3742356128,-11.8721618652));
#97403=CARTESIAN_POINT('Origin',(0.,-19.3742356128,0.473661560394));
#97404=CARTESIAN_POINT('',(-4.2,-19.3742356128,-7.3013690143));
#97405=CARTESIAN_POINT('',(-3.91586593048,-19.3742356128,-7.3013690143));
#97406=CARTESIAN_POINT('',(-6.,-19.3742356128,-5.5013690143));
#97407=CARTESIAN_POINT('Origin',(-4.2,-19.3742356128,-5.5013690143));
#97408=CARTESIAN_POINT('',(-6.,-19.3742356128,-3.77162994903));
#97409=CARTESIAN_POINT('',(-6.,-19.3742356128,-4.63649948183));
#97410=CARTESIAN_POINT('',(-6.,-19.3742356128,4.71895306982));
#97411=CARTESIAN_POINT('Origin',(0.,-19.3742356128,0.473661560394));
#97412=CARTESIAN_POINT('',(-6.,-19.3742356128,6.1986309857));
#97413=CARTESIAN_POINT('',(-6.,-19.3742356128,5.45879202751));
#97414=CARTESIAN_POINT('',(-5.60798767447,-19.3742356128,7.32004558724));
#97415=CARTESIAN_POINT('Origin',(-4.2,-19.3742356128,6.1986309857));
#97416=CARTESIAN_POINT('',(-7.62360441819,-19.3742356128,4.96845362177));
#97417=CARTESIAN_POINT('Origin',(0.,-19.3742356128,0.473661560394));
#97418=CARTESIAN_POINT('',(-9.82022628685,-19.3742356128,4.96845362177));
#97419=CARTESIAN_POINT('',(-8.72191535252,-19.3742356128,4.96845362177));
#97420=CARTESIAN_POINT('',(-5.98285024331,-19.3742356128,-8.51775117433));
#97421=CARTESIAN_POINT('Origin',(0.,-19.3742356128,0.473661560394));
#97422=CARTESIAN_POINT('',(-5.17999195052,-19.3742356128,-10.0163199637));
#97423=CARTESIAN_POINT('Origin',(-6.97999195052,-19.3742356128,-10.0163199635));
#97424=CARTESIAN_POINT('',(-5.17999195052,-19.3742356128,-12.4003392757));
#97425=CARTESIAN_POINT('',(-5.17999195052,-19.3742356128,-11.2083296197));
#97426=CARTESIAN_POINT('',(-4.10871050222,-19.3742356128,-12.4074193595));
#97427=CARTESIAN_POINT('Origin',(-4.65570820166,-19.3742356128,-14.1222935581));
#97428=CARTESIAN_POINT('',(-3.03907448041,-19.3742356128,-12.7008507251));
#97429=CARTESIAN_POINT('Origin',(0.,-19.3742356128,0.473661560394));
#97430=CARTESIAN_POINT('',(-1.95746548311,-19.3742356128,-13.4393118415));
#97431=CARTESIAN_POINT('Origin',(-3.4436702163,-19.3742356128,-14.4547898034));
#97432=CARTESIAN_POINT('',(1.95746548311,-19.3742356128,-13.4393118415));
#97433=CARTESIAN_POINT('Origin',(0.,-19.3742356128,0.473661560394));
#97434=CARTESIAN_POINT('',(3.03907448041,-19.3742356128,-12.7008507251));
#97435=CARTESIAN_POINT('Origin',(3.4436702163,-19.3742356128,-14.4547898034));
#97436=CARTESIAN_POINT('',(4.16144704355,-19.3742356128,-12.3904787591));
#97437=CARTESIAN_POINT('Origin',(0.,-19.3742356128,0.473661560394));
#97438=CARTESIAN_POINT('',(5.17999195052,-19.3742356128,-12.3640705239));
#97439=CARTESIAN_POINT('Origin',(4.71546562382,-19.3742356128,-14.1030976346));
#97440=CARTESIAN_POINT('',(5.17999195052,-19.3742356128,-10.0163199635));
#97441=CARTESIAN_POINT('',(5.17999195052,-19.3742356128,-11.1901952438));
#97442=CARTESIAN_POINT('',(5.98285024331,-19.3742356128,-8.51775117433));
#97443=CARTESIAN_POINT('Origin',(6.97999195052,-19.3742356128,-10.0163199635));
#97444=CARTESIAN_POINT('',(9.82022628685,-19.3742356128,4.96845362177));
#97445=CARTESIAN_POINT('Origin',(0.,-19.3742356128,0.473661560394));
#97446=CARTESIAN_POINT('',(7.62360441819,-19.3742356128,4.96845362177));
#97447=CARTESIAN_POINT('',(8.72191535252,-19.3742356128,4.96845362177));
#97448=CARTESIAN_POINT('',(5.60798767447,-19.3742356128,7.32004558724));
#97449=CARTESIAN_POINT('Origin',(0.,-19.3742356128,0.473661560394));
#97450=CARTESIAN_POINT('',(6.,-19.3742356128,6.1986309857));
#97451=CARTESIAN_POINT('Origin',(4.2,-19.3742356128,6.1986309857));
#97452=CARTESIAN_POINT('',(6.,-19.3742356128,4.71895306982));
#97453=CARTESIAN_POINT('',(6.,-19.3742356128,5.45879202751));
#97454=CARTESIAN_POINT('',(6.,-19.3742356128,-3.77162994903));
#97455=CARTESIAN_POINT('Origin',(0.,-19.3742356128,0.473661560394));
#97456=CARTESIAN_POINT('',(6.,-19.3742356128,-5.5013690143));
#97457=CARTESIAN_POINT('',(6.,-19.3742356128,-4.63649948183));
#97458=CARTESIAN_POINT('',(4.20000000006,-19.3742356128,-7.3013690143));
#97459=CARTESIAN_POINT('Origin',(4.2,-19.3742356128,-5.5013690143));
#97460=CARTESIAN_POINT('',(3.91586593048,-19.3742356128,-7.3013690143));
#97461=CARTESIAN_POINT('Origin',(0.,-20.2352955315,-4.4019615652));
#97462=CARTESIAN_POINT('',(3.93695199971652,-18.7782619834169,-5.99493429549677));
#97463=CARTESIAN_POINT('',(-3.93695210731,-18.7782622649,-5.99493430976));
#97464=CARTESIAN_POINT('Origin',(-1.50990331349E-14,-20.2352955315,-5.99493430976));
#97465=CARTESIAN_POINT('Ctrl Pts',(-3.9369521072875,-18.7782622649083,-5.9949343097509));
#97466=CARTESIAN_POINT('Ctrl Pts',(-3.9705399999975,-18.8690178544819,-5.9949343023535));
#97467=CARTESIAN_POINT('Ctrl Pts',(-4.0019605374177,-18.9602724232578,-5.99192992634488));
#97468=CARTESIAN_POINT('Ctrl Pts',(-4.03081052657067,-19.0520074442237,
-5.98704698577112));
#97469=CARTESIAN_POINT('Ctrl Pts',(-4.04074578399551,-19.0835988269218,
-5.98536541593297));
#97470=CARTESIAN_POINT('Ctrl Pts',(-4.05037639795643,-19.1152474735558,
-5.98346074163699));
#97471=CARTESIAN_POINT('Ctrl Pts',(-4.05968616233678,-19.1469533287217,
-5.9813790244995));
#97472=CARTESIAN_POINT('Ctrl Pts',(4.05968610441,-19.1469533038,-5.98137915695));
#97473=CARTESIAN_POINT('Ctrl Pts',(4.03788343644,-19.0727011908,-5.98625455018));
#97474=CARTESIAN_POINT('Ctrl Pts',(4.01461432289,-18.9987108858,-5.9903211697));
#97475=CARTESIAN_POINT('Ctrl Pts',(3.98996106595,-18.9249385271,-5.99330264064));
#97476=CARTESIAN_POINT('Ctrl Pts',(3.96404157784,-18.8514591938,-5.99493417698));
#97477=CARTESIAN_POINT('Ctrl Pts',(3.93695201003,-18.7782619796,-5.99493428923));
#97478=CARTESIAN_POINT('Origin',(0.,-4.67423561284,0.473661560394));
#97479=CARTESIAN_POINT('',(4.2,-4.67423561284,6.4986309857));
#97480=CARTESIAN_POINT('Origin',(4.2,-4.67423561284,6.1986309857));
#97481=CARTESIAN_POINT('',(-4.2,-4.67423561284,6.4986309857));
#97482=CARTESIAN_POINT('',(0.,-4.67423561284,6.4986309857));
#97483=CARTESIAN_POINT('',(-4.5,-4.67423561284,6.1986309857));
#97484=CARTESIAN_POINT('Origin',(-4.2,-4.67423561284,6.1986309857));
#97485=CARTESIAN_POINT('',(-4.5,-4.67423561284,3.49012794495));
#97486=CARTESIAN_POINT('',(-4.5,-4.67423561284,4.84437946532));
#97487=CARTESIAN_POINT('',(-5.44794311523,-4.67423561284,3.49012794495));
#97488=CARTESIAN_POINT('',(-4.97448577881,-4.67423561284,3.49012794495));
#97489=CARTESIAN_POINT('',(-5.44794311523,-4.67423561284,-2.54280482416));
#97490=CARTESIAN_POINT('',(-5.44794311523,-4.67423561284,1.98189475267));
#97491=CARTESIAN_POINT('',(-4.5,-4.67423561284,-2.54280482416));
#97492=CARTESIAN_POINT('',(-4.97448577881,-4.67423561284,-2.54280482416));
#97493=CARTESIAN_POINT('',(-4.5,-4.67423561284,-5.5013690143));
#97494=CARTESIAN_POINT('',(-4.5,-4.67423561284,-4.02208691923));
#97495=CARTESIAN_POINT('',(-4.2,-4.67423561284,-5.8013690143));
#97496=CARTESIAN_POINT('Origin',(-4.2,-4.67423561284,-5.5013690143));
#97497=CARTESIAN_POINT('',(4.2,-4.67423561284,-5.8013690143));
#97498=CARTESIAN_POINT('',(0.,-4.67423561284,-5.8013690143));
#97499=CARTESIAN_POINT('',(4.5,-4.67423561284,-5.5013690143));
#97500=CARTESIAN_POINT('Origin',(4.2,-4.67423561284,-5.5013690143));
#97501=CARTESIAN_POINT('',(4.5,-4.67423561284,0.348630985699));
#97502=CARTESIAN_POINT('Origin',(0.,-4.67423561284,0.473661560394));
#97503=CARTESIAN_POINT('',(-8.40228522294909E-15,-4.67423561284,9.323661560394));
#97504=CARTESIAN_POINT('Origin',(0.,-4.67423561284,0.473661560394));
#97505=CARTESIAN_POINT('Origin',(0.,-4.67423561284,0.473661560394));
#97506=CARTESIAN_POINT('Origin',(-4.5,-4.67423561284,6.4986309857));
#97507=CARTESIAN_POINT('',(-4.5,-19.0742356128,-5.5013690143));
#97508=CARTESIAN_POINT('',(-4.5,-19.0742356128,6.1986309857));
#97509=CARTESIAN_POINT('',(-4.5,-19.0742356128,-2.12633843961));
#97510=CARTESIAN_POINT('',(-4.5,-13.6742356128,-5.5013690143));
#97511=CARTESIAN_POINT('',(-4.5,-14.0742356128,-2.54280482416));
#97512=CARTESIAN_POINT('',(-4.5,-9.37423561284,-2.54280482416));
#97513=CARTESIAN_POINT('',(-4.5,-14.0742356128,3.49012794495));
#97514=CARTESIAN_POINT('',(-4.5,-14.0742356128,1.98189475267));
#97515=CARTESIAN_POINT('',(-4.5,-9.37423561284,3.49012794495));
#97516=CARTESIAN_POINT('',(-4.5,-13.6742356128,6.1986309857));
#97517=CARTESIAN_POINT('Origin',(7.85,-9.17423561284,0.473661560394));
#97518=CARTESIAN_POINT('',(-8.85,-7.67423561284,0.473661560394));
#97519=CARTESIAN_POINT('',(-8.78621078736448,-10.2348957846198,1.53432173217382));
#97520=CARTESIAN_POINT('Ctrl Pts',(-8.85,-7.67423561284,0.473661560394));
#97521=CARTESIAN_POINT('Ctrl Pts',(-8.85,-7.67423561284,0.662394292391));
#97522=CARTESIAN_POINT('Ctrl Pts',(-8.84334932535928,-7.71202837241176,
0.863460154972133));
#97523=CARTESIAN_POINT('Ctrl Pts',(-8.81931354586398,-7.86522295898186,
1.23292358106269));
#97524=CARTESIAN_POINT('Ctrl Pts',(-8.80226283219622,-7.98060481275496,
1.4013511038686));
#97525=CARTESIAN_POINT('Ctrl Pts',(-8.77015828355848,-8.24654987137926,
1.66729616249291));
#97526=CARTESIAN_POINT('Ctrl Pts',(-8.75299937723619,-8.41497576333756,
1.78267503425714));
#97527=CARTESIAN_POINT('Ctrl Pts',(-8.72871516126698,-8.78443358162711,
1.93586745610213));
#97528=CARTESIAN_POINT('Ctrl Pts',(-8.72195505606398,-8.98549748442973,
1.973661560394));
#97529=CARTESIAN_POINT('Ctrl Pts',(-8.72195505606398,-9.36297374125027,
1.973661560394));
#97530=CARTESIAN_POINT('Ctrl Pts',(-8.72871516126698,-9.5640376440529,1.93586745610213));
#97531=CARTESIAN_POINT('Ctrl Pts',(-8.75299937723619,-9.93349546234244,
1.78267503425714));
#97532=CARTESIAN_POINT('Ctrl Pts',(-8.77015828355847,-10.1019213543007,
1.6672961624929));
#97533=CARTESIAN_POINT('Ctrl Pts',(-8.78621078736448,-10.2348957846198,
1.53432173217382));
#97534=CARTESIAN_POINT('Ctrl Pts',(-8.78621078736448,-10.2348957846198,
1.53432173217382));
#97535=CARTESIAN_POINT('Ctrl Pts',(-8.80226283219622,-10.367866412925,1.4013511038686));
#97536=CARTESIAN_POINT('Ctrl Pts',(-8.81931354586398,-10.4832482666981,
1.23292358106269));
#97537=CARTESIAN_POINT('Ctrl Pts',(-8.84334932535928,-10.6364428532682,
0.863460154972134));
#97538=CARTESIAN_POINT('Ctrl Pts',(-8.85,-10.67423561284,0.662394292390999));
#97539=CARTESIAN_POINT('Ctrl Pts',(-8.85,-10.67423561284,0.284928828397001));
#97540=CARTESIAN_POINT('Ctrl Pts',(-8.84334932535928,-10.6364428532682,
0.083862965815866));
#97541=CARTESIAN_POINT('Ctrl Pts',(-8.81931354586398,-10.4832482666981,
-0.285600460274688));
#97542=CARTESIAN_POINT('Ctrl Pts',(-8.80226283219622,-10.367866412925,-0.4540279830806));
#97543=CARTESIAN_POINT('Ctrl Pts',(-8.77015828355847,-10.1019213543007,
-0.719973041704904));
#97544=CARTESIAN_POINT('Ctrl Pts',(-8.75299937723619,-9.93349546234244,
-0.835351913469144));
#97545=CARTESIAN_POINT('Ctrl Pts',(-8.72871516126698,-9.5640376440529,-0.988544335314129));
#97546=CARTESIAN_POINT('Ctrl Pts',(-8.72195505606398,-9.36297374125027,
-1.026338439606));
#97547=CARTESIAN_POINT('Ctrl Pts',(-8.72195505606398,-9.17423561284,-1.026338439606));
#97548=CARTESIAN_POINT('Ctrl Pts',(-8.72195505606398,-8.98549748442973,
-1.026338439606));
#97549=CARTESIAN_POINT('Ctrl Pts',(-8.72871516126698,-8.78443358162711,
-0.988544335314129));
#97550=CARTESIAN_POINT('Ctrl Pts',(-8.75299937723619,-8.41497576333756,
-0.835351913469143));
#97551=CARTESIAN_POINT('Ctrl Pts',(-8.77015828355848,-8.24654987137926,
-0.719973041704905));
#97552=CARTESIAN_POINT('Ctrl Pts',(-8.80226283219622,-7.98060481275496,
-0.4540279830806));
#97553=CARTESIAN_POINT('Ctrl Pts',(-8.81931354586398,-7.86522295898186,
-0.285600460274688));
#97554=CARTESIAN_POINT('Ctrl Pts',(-8.84334932535928,-7.71202837241176,
0.0838629658158672));
#97555=CARTESIAN_POINT('Ctrl Pts',(-8.85,-7.67423561284,0.284928828397001));
#97556=CARTESIAN_POINT('Ctrl Pts',(-8.85,-7.67423561284,0.473661560394));
#97557=CARTESIAN_POINT('',(-5.44794311523,-10.2348957846198,1.53432173217382));
#97558=CARTESIAN_POINT('',(7.85,-10.2348957846198,1.53432173217382));
#97559=CARTESIAN_POINT('Origin',(-5.44794311523,-9.17423561284,0.473661560394));
#97560=CARTESIAN_POINT('Origin',(-6.61089801788,-14.9244482822,0.473661560394));
#97561=CARTESIAN_POINT('',(-6.61089801788,-14.9244482822,-5.41008957278));
#97562=CARTESIAN_POINT('',(-6.61089801788,-9.92423561284,-5.41008957278));
#97563=CARTESIAN_POINT('',(-6.61089801788,-12.0242356128,-5.41008957278));
#97564=CARTESIAN_POINT('',(-6.61089801788,-14.9244482822,-0.276338439606));
#97565=CARTESIAN_POINT('',(-6.61089801788,-14.9244482822,-2.84321400619));
#97566=CARTESIAN_POINT('',(-6.61089801788,-12.6613939106,-0.276338439606));
#97567=CARTESIAN_POINT('',(-6.61089801788,-13.7929210964,-0.276338439606));
#97568=CARTESIAN_POINT('',(-6.61089801788,-10.2242096029,-2.07631242966));
#97569=CARTESIAN_POINT('Origin',(-6.61089801788,-10.2242096029,0.473661560394));
#97570=CARTESIAN_POINT('',(-6.61089801788,-9.92423561284,-2.07631242966));
#97571=CARTESIAN_POINT('',(-6.61089801788,-10.0742226079,-2.07631242966));
#97572=CARTESIAN_POINT('',(-6.61089801788,-9.92423561284,-3.74320100122));
#97573=CARTESIAN_POINT('Origin',(4.,-9.92423561284,10.9094726032));
#97574=CARTESIAN_POINT('',(-8.47467596136,-9.92423561284,-2.07631242966));
#97575=CARTESIAN_POINT('',(-7.54278698962,-9.92423561284,-2.07631242966));
#97576=CARTESIAN_POINT('Origin',(0.,-9.92423561284,0.473661560394));
#97577=CARTESIAN_POINT('Origin',(9.7,-9.17423561284,-2.07631242966));
#97578=CARTESIAN_POINT('',(-8.47467596136,-10.2242096029,-2.07631242966));
#97579=CARTESIAN_POINT('',(-8.47467596136,-9.81495241206,-2.07631242966));
#97580=CARTESIAN_POINT('',(7.23999999989,-10.2242096029,-2.07631242966));
#97581=CARTESIAN_POINT('Origin',(7.23999999989,-10.2242096029,0.473661560394));
#97582=CARTESIAN_POINT('',(-8.81816307332978,-12.6613939105328,-0.276338439790844));
#97583=CARTESIAN_POINT('Ctrl Pts',(-8.81816307399792,-12.6613939105698,
-0.276338439859058));
#97584=CARTESIAN_POINT('Ctrl Pts',(-8.81159014191855,-12.6376118819527,
-0.353620022433216));
#97585=CARTESIAN_POINT('Ctrl Pts',(-8.80407126472156,-12.6100918009648,
-0.429935532759619));
#97586=CARTESIAN_POINT('Ctrl Pts',(-8.76084293562039,-12.4486247941201,
-0.818571700939171));
#97587=CARTESIAN_POINT('Ctrl Pts',(-8.71126631028426,-12.2526596929331,
-1.10409615000023));
#97588=CARTESIAN_POINT('Ctrl Pts',(-8.61746290023769,-11.8019105710455,
-1.55484527188781));
#97589=CARTESIAN_POINT('Ctrl Pts',(-8.56695493619419,-11.516409326613,-1.75076635383017));
#97590=CARTESIAN_POINT('Ctrl Pts',(-8.49497179593289,-10.8887452246525,
-2.01154492600502));
#97591=CARTESIAN_POINT('Ctrl Pts',(-8.47467596136091,-10.5464102971449,
-2.076312429656));
#97592=CARTESIAN_POINT('Ctrl Pts',(-8.47467596136091,-10.2242096029,-2.076312429656));
#97593=CARTESIAN_POINT('',(-7.71453053854,-12.6613939106,-0.276338439606));
#97594=CARTESIAN_POINT('Origin',(4.,-11.2955559564,-0.276338439606));
#97595=CARTESIAN_POINT('',(-8.81816307402,-14.9244482822,-0.276338439606));
#97596=CARTESIAN_POINT('',(-8.81816307402,-9.81495241206,-0.276338439606));
#97597=CARTESIAN_POINT('',(-7.71453054595,-14.9244482822,-0.276338439606));
#97598=CARTESIAN_POINT('Origin',(13.7258691788,-14.9244482822,0.473661560394));
#97599=CARTESIAN_POINT('Origin',(0.,-14.9244482822,0.473661560394));
#97600=CARTESIAN_POINT('Origin',(6.61089801788,-5.78170707891,0.473661560394));
#97601=CARTESIAN_POINT('',(-8.81816307402,-5.78170707891,-0.276338439606));
#97602=CARTESIAN_POINT('',(-6.61089801788,-5.78170707891,-5.41008957278));
#97603=CARTESIAN_POINT('Origin',(0.,-5.78170707891,0.473661560394));
#97604=CARTESIAN_POINT('',(-6.61089801788,-5.78170707891,-0.276338439606));
#97605=CARTESIAN_POINT('',(-6.61089801788,-5.78170707891,-2.84321400619));
#97606=CARTESIAN_POINT('',(-7.71453054595,-5.78170707891,-0.276338439606));
#97607=CARTESIAN_POINT('Origin',(-6.61089801788,-14.9244482822,0.473661560394));
#97608=CARTESIAN_POINT('',(-6.61089801788,-8.42423561284,-5.41008957278));
#97609=CARTESIAN_POINT('',(-6.61089801788,-12.0242356128,-5.41008957278));
#97610=CARTESIAN_POINT('',(-6.61089801788,-8.42423561284,-1.963549961));
#97611=CARTESIAN_POINT('',(-6.61089801788,-8.42423561284,-3.68681976689));
#97612=CARTESIAN_POINT('',(-6.61089801788,-6.73702409145,-0.276338439606));
#97613=CARTESIAN_POINT('Origin',(-6.61089801788,-9.17423561284,0.473661560394));
#97614=CARTESIAN_POINT('',(-6.61089801788,-6.25936558518,-0.276338439606));
#97615=CARTESIAN_POINT('Origin',(4.,-11.2955559564,-0.276338439606));
#97616=CARTESIAN_POINT('',(-8.81816307402,-6.73702409145,-0.276338439606));
#97617=CARTESIAN_POINT('',(-8.81816307402,-9.81495241206,-0.276338439606));
#97618=CARTESIAN_POINT('',(7.85,-6.73702409145,-0.276338439606));
#97619=CARTESIAN_POINT('Origin',(7.85,-9.17423561284,0.473661560394));
#97620=CARTESIAN_POINT('',(-8.50779054749,-8.42423561284,-1.963549961));
#97621=CARTESIAN_POINT('',(-7.55934428269,-8.42423561284,-1.963549961));
#97622=CARTESIAN_POINT('Ctrl Pts',(-8.50779054749224,-8.42423561284108,
-1.96354996099712));
#97623=CARTESIAN_POINT('Ctrl Pts',(-8.51460395755545,-8.34694619186505,
-1.93976578583499));
#97624=CARTESIAN_POINT('Ctrl Pts',(-8.52238203382313,-8.27062509791715,
-1.91224351726085));
#97625=CARTESIAN_POINT('Ctrl Pts',(-8.5669490755189,-7.88202266221689,-1.75078901559462));
#97626=CARTESIAN_POINT('Ctrl Pts',(-8.61745809932542,-7.59651853184558,
-1.55486594266297));
#97627=CARTESIAN_POINT('Ctrl Pts',(-8.71126345553147,-7.14576485501596,
-1.10411226583335));
#97628=CARTESIAN_POINT('Ctrl Pts',(-8.76084110174091,-6.94979776054387,
-0.818584929648812));
#97629=CARTESIAN_POINT('Ctrl Pts',(-8.80407059609266,-6.78832806722135,
-0.429942320036869));
#97630=CARTESIAN_POINT('Ctrl Pts',(-8.811589850943,-6.76080690738505,-0.353623443619236));
#97631=CARTESIAN_POINT('Ctrl Pts',(-8.81816307401943,-6.73702409144926,
-0.276338439606178));
#97632=CARTESIAN_POINT('Origin',(4.,-8.42423561284,10.9094726032));
#97633=CARTESIAN_POINT('Origin',(0.,-8.42423561284,0.473661560394));
#97634=CARTESIAN_POINT('Origin',(-6.61089801788,-14.9244482822,0.473661560394));
#97635=CARTESIAN_POINT('',(-6.61089801788,-8.42423561284,6.35741269357));
#97636=CARTESIAN_POINT('',(-6.61089801788,-5.78170707891,6.35741269357));
#97637=CARTESIAN_POINT('',(-6.61089801788,-12.0242356128,6.35741269357));
#97638=CARTESIAN_POINT('',(-6.61089801788,-5.78170707891,1.22366156039));
#97639=CARTESIAN_POINT('',(-6.61089801788,-5.78170707891,3.79053712698));
#97640=CARTESIAN_POINT('',(-6.61089801788,-6.73702409145,1.22366156039));
#97641=CARTESIAN_POINT('',(-6.61089801788,-6.25936558518,1.22366156039));
#97642=CARTESIAN_POINT('',(-6.61089801788,-8.42423561284,2.91087308178));
#97643=CARTESIAN_POINT('Origin',(-6.61089801788,-9.17423561284,0.473661560394));
#97644=CARTESIAN_POINT('',(-6.61089801788,-8.42423561284,4.63414288768));
#97645=CARTESIAN_POINT('Origin',(4.,-8.42423561284,10.9094726032));
#97646=CARTESIAN_POINT('',(-8.50779054749,-8.42423561284,2.91087308178));
#97647=CARTESIAN_POINT('Origin',(0.,-8.42423561284,0.473661560394));
#97648=CARTESIAN_POINT('',(7.85,-8.42423561284,2.91087308178));
#97649=CARTESIAN_POINT('Origin',(7.85,-9.17423561284,0.473661560394));
#97650=CARTESIAN_POINT('',(-8.81816307402,-6.73702409145,1.22366156039));
#97651=CARTESIAN_POINT('',(-7.71453054595,-6.73702409145,1.22366156039));
#97652=CARTESIAN_POINT('Ctrl Pts',(-8.50779054749244,-8.42423561283885,
2.91087308178444));
#97653=CARTESIAN_POINT('Ctrl Pts',(-8.5146039575556,-8.34694619186358,2.88708890662246));
#97654=CARTESIAN_POINT('Ctrl Pts',(-8.52238203382321,-8.27062509791643,
2.85956663804855));
#97655=CARTESIAN_POINT('Ctrl Pts',(-8.5669490755189,-7.88202266221689,2.69811213638263));
#97656=CARTESIAN_POINT('Ctrl Pts',(-8.61745809932542,-7.59651853184558,
2.50218906345097));
#97657=CARTESIAN_POINT('Ctrl Pts',(-8.71126345553147,-7.14576485501596,
2.05143538662135));
#97658=CARTESIAN_POINT('Ctrl Pts',(-8.76084110174091,-6.94979776054387,
1.76590805043681));
#97659=CARTESIAN_POINT('Ctrl Pts',(-8.80407059609279,-6.78832806722086,
1.3772654408237));
#97660=CARTESIAN_POINT('Ctrl Pts',(-8.81158985094324,-6.76080690738419,
1.30094656440485));
#97661=CARTESIAN_POINT('Ctrl Pts',(-8.81816307401973,-6.73702409144815,
1.22366156039055));
#97662=CARTESIAN_POINT('Origin',(4.,-2.81495241206,1.22366156039));
#97663=CARTESIAN_POINT('',(-8.81816307402,-5.78170707891,1.22366156039));
#97664=CARTESIAN_POINT('',(-7.71453054595,-5.78170707891,1.22366156039));
#97665=CARTESIAN_POINT('',(-8.81816307402,-9.81495241206,1.22366156039));
#97666=CARTESIAN_POINT('Origin',(6.61089801788,-5.78170707891,0.473661560394));
#97667=CARTESIAN_POINT('Origin',(0.,-5.78170707891,0.473661560394));
#97668=CARTESIAN_POINT('Origin',(13.7258691788,-14.9244482822,0.473661560394));
#97669=CARTESIAN_POINT('',(-8.81816307402,-14.9244482822,1.22366156039));
#97670=CARTESIAN_POINT('',(-6.61089801788,-14.9244482822,6.35741269357));
#97671=CARTESIAN_POINT('Origin',(0.,-14.9244482822,0.473661560394));
#97672=CARTESIAN_POINT('',(-6.61089801788,-14.9244482822,1.22366156039));
#97673=CARTESIAN_POINT('',(-6.61089801788,-14.9244482822,3.79053712698));
#97674=CARTESIAN_POINT('',(-7.71453054595,-14.9244482822,1.22366156039));
#97675=CARTESIAN_POINT('Origin',(-6.61089801788,-14.9244482822,0.473661560394));
#97676=CARTESIAN_POINT('',(-6.61089801788,-9.92423561284,6.35741269357));
#97677=CARTESIAN_POINT('',(-6.61089801788,-12.0242356128,6.35741269357));
#97678=CARTESIAN_POINT('',(-6.61089801788,-9.92423561284,3.02363555044));
#97679=CARTESIAN_POINT('',(-6.61089801788,-9.92423561284,4.69052412201));
#97680=CARTESIAN_POINT('',(-6.61089801788,-10.2242096029,3.02363555044));
#97681=CARTESIAN_POINT('',(-6.61089801788,-10.0742226079,3.02363555044));
#97682=CARTESIAN_POINT('',(-6.61089801788,-12.6613939106,1.22366156039));
#97683=CARTESIAN_POINT('Origin',(-6.61089801788,-10.2242096029,0.473661560394));
#97684=CARTESIAN_POINT('',(-6.61089801788,-13.7929210964,1.22366156039));
#97685=CARTESIAN_POINT('Origin',(4.,-2.81495241206,1.22366156039));
#97686=CARTESIAN_POINT('',(-8.81816307334515,-12.6613939101212,1.22366156090261));
#97687=CARTESIAN_POINT('',(7.23999999989,-12.6613939106,1.22366156039));
#97688=CARTESIAN_POINT('',(-8.81816307402,-9.81495241206,1.22366156039));
#97689=CARTESIAN_POINT('Origin',(7.23999999989,-10.2242096029,0.473661560394));
#97690=CARTESIAN_POINT('',(-8.47467596136,-10.2242096029,3.02363555044));
#97691=CARTESIAN_POINT('Ctrl Pts',(-8.47467596136091,-10.2242096029,3.023635550444));
#97692=CARTESIAN_POINT('Ctrl Pts',(-8.47467596136091,-10.5464102971449,
3.023635550444));
#97693=CARTESIAN_POINT('Ctrl Pts',(-8.49497179593289,-10.8887452246525,
2.95886804679302));
#97694=CARTESIAN_POINT('Ctrl Pts',(-8.56695493619419,-11.516409326613,2.69808947461818));
#97695=CARTESIAN_POINT('Ctrl Pts',(-8.61746290023769,-11.8019105710455,
2.50216839267581));
#97696=CARTESIAN_POINT('Ctrl Pts',(-8.71126631028426,-12.2526596929331,
2.05141927078824));
#97697=CARTESIAN_POINT('Ctrl Pts',(-8.76084293562039,-12.4486247941201,
1.76589482172717));
#97698=CARTESIAN_POINT('Ctrl Pts',(-8.80407126470694,-12.6100918009102,
1.37725865367903));
#97699=CARTESIAN_POINT('Ctrl Pts',(-8.81159014189213,-12.637611881856,1.30094314348955));
#97700=CARTESIAN_POINT('Ctrl Pts',(-8.81816307396325,-12.6613939104444,
1.22366156105464));
#97701=CARTESIAN_POINT('',(-7.54278698962,-10.2242096029,3.02363555044));
#97702=CARTESIAN_POINT('Origin',(9.7,-9.17423561284,3.02363555044));
#97703=CARTESIAN_POINT('',(-8.47467596136,-9.92423561284,3.02363555044));
#97704=CARTESIAN_POINT('',(-8.47467596136,-9.81495241206,3.02363555044));
#97705=CARTESIAN_POINT('',(-7.54278698962,-9.92423561284,3.02363555044));
#97706=CARTESIAN_POINT('Origin',(4.,-9.92423561284,10.9094726032));
#97707=CARTESIAN_POINT('Origin',(0.,-9.92423561284,0.473661560394));
#97708=CARTESIAN_POINT('Origin',(13.7258691788,-16.4244482822,0.473661560394));
#97709=CARTESIAN_POINT('',(-6.,-16.4244482822,4.71895306982));
#97710=CARTESIAN_POINT('',(-6.,-16.4244482822,-3.77162994903));
#97711=CARTESIAN_POINT('Origin',(0.,-16.4244482822,0.473661560394));
#97712=CARTESIAN_POINT('',(-6.,-16.4244482822,0.348630985699));
#97713=CARTESIAN_POINT('Origin',(13.7258691788,-16.4244482822,0.473661560394));
#97714=CARTESIAN_POINT('',(6.,-16.4244482822,-3.77162994903));
#97715=CARTESIAN_POINT('',(6.,-16.4244482822,4.71895306982));
#97716=CARTESIAN_POINT('Origin',(0.,-16.4244482822,0.473661560394));
#97717=CARTESIAN_POINT('',(6.,-16.4244482822,0.348630985699));
#97718=CARTESIAN_POINT('Origin',(0.,-12.0242356128,0.473661560394));
#97719=CARTESIAN_POINT('',(6.,-12.7742356128,4.71895306982));
#97720=CARTESIAN_POINT('',(6.,-12.7742356128,-3.77162994903));
#97721=CARTESIAN_POINT('Origin',(0.,-12.0242356128,0.473661560394));
#97722=CARTESIAN_POINT('',(-6.,-12.7742356128,4.71895306982));
#97723=CARTESIAN_POINT('',(-6.,-12.7742356128,-3.77162994903));
#97724=CARTESIAN_POINT('Origin',(0.,-18.1742356128,0.473661560394));
#97725=CARTESIAN_POINT('',(-4.84699160505,-18.1742356128,7.87833389485));
#97726=CARTESIAN_POINT('',(4.84699160505,-18.1742356128,7.87833389485));
#97727=CARTESIAN_POINT('Origin',(0.,-18.1742356128,0.473661560394));
#97728=CARTESIAN_POINT('',(-4.2,-18.1742356128,7.9986309857));
#97729=CARTESIAN_POINT('Origin',(-4.2,-18.1742356128,6.1986309857));
#97730=CARTESIAN_POINT('',(4.2,-18.1742356128,7.9986309857));
#97731=CARTESIAN_POINT('',(0.,-18.1742356128,7.9986309857));
#97732=CARTESIAN_POINT('Origin',(4.2,-18.1742356128,6.1986309857));
#97733=CARTESIAN_POINT('Origin',(-6.,-4.67423561284,6.4986309857));
#97734=CARTESIAN_POINT('',(-6.,-19.3742356128,0.473661560394));
#97735=CARTESIAN_POINT('Origin',(6.,-4.67423561284,6.4986309857));
#97736=CARTESIAN_POINT('',(6.,-19.3742356128,0.473661560394));
#97737=CARTESIAN_POINT('Origin',(0.,-18.0242356128,0.473661560394));
#97738=CARTESIAN_POINT('',(-4.84699160505,-19.3742356128,7.87833389485));
#97739=CARTESIAN_POINT('',(4.84699160505,-19.3742356128,7.87833389485));
#97740=CARTESIAN_POINT('Origin',(0.,-19.3742356128,0.473661560394));
#97741=CARTESIAN_POINT('',(-4.84699160505,-12.7742356128,7.87833389485));
#97742=CARTESIAN_POINT('',(4.84699160505,-12.7742356128,7.87833389485));
#97743=CARTESIAN_POINT('Origin',(4.2,-13.6742356128,6.1986309857));
#97744=CARTESIAN_POINT('',(4.2,-19.3742356128,7.9986309857));
#97745=CARTESIAN_POINT('Origin',(4.2,-19.3742356128,6.1986309857));
#97746=CARTESIAN_POINT('',(4.2,-12.7742356128,7.9986309857));
#97747=CARTESIAN_POINT('Origin',(0.,-4.67423561284,7.9986309857));
#97748=CARTESIAN_POINT('',(-4.2,-19.3742356128,7.9986309857));
#97749=CARTESIAN_POINT('',(-4.2,-12.7742356128,7.9986309857));
#97750=CARTESIAN_POINT('',(0.,-19.3742356128,7.9986309857));
#97751=CARTESIAN_POINT('Origin',(-4.2,-13.6742356128,6.1986309857));
#97752=CARTESIAN_POINT('Origin',(-4.2,-19.3742356128,6.1986309857));
#97753=CARTESIAN_POINT('Origin',(7.85,-9.17423561284,0.473661560394));
#97754=CARTESIAN_POINT('',(4.5,-10.2348957846198,1.53432173217382));
#97755=CARTESIAN_POINT('Origin',(4.5,-9.17423561284,0.473661560394));
#97756=CARTESIAN_POINT('',(8.78621078736448,-10.2348957846198,1.53432173217382));
#97757=CARTESIAN_POINT('',(7.85,-10.2348957846198,1.53432173217382));
#97758=CARTESIAN_POINT('',(8.85,-10.6742356128,0.473661560394));
#97759=CARTESIAN_POINT('Ctrl Pts',(8.78621078736448,-10.2348957846198,1.53432173217382));
#97760=CARTESIAN_POINT('Ctrl Pts',(8.80226283219622,-10.367866412925,1.4013511038686));
#97761=CARTESIAN_POINT('Ctrl Pts',(8.81931354586398,-10.4832482666981,1.23292358106269));
#97762=CARTESIAN_POINT('Ctrl Pts',(8.84334932535928,-10.6364428532682,0.863460154972133));
#97763=CARTESIAN_POINT('Ctrl Pts',(8.85,-10.67423561284,0.662394292390999));
#97764=CARTESIAN_POINT('Ctrl Pts',(8.85,-10.67423561284,0.473661560394));
#97765=CARTESIAN_POINT('Ctrl Pts',(8.85,-10.67423561284,0.473661560394));
#97766=CARTESIAN_POINT('Ctrl Pts',(8.85,-10.67423561284,0.284928828397001));
#97767=CARTESIAN_POINT('Ctrl Pts',(8.84334932535928,-10.6364428532682,0.0838629658158659));
#97768=CARTESIAN_POINT('Ctrl Pts',(8.81931354586398,-10.4832482666981,-0.285600460274688));
#97769=CARTESIAN_POINT('Ctrl Pts',(8.80226283219622,-10.367866412925,-0.454027983080601));
#97770=CARTESIAN_POINT('Ctrl Pts',(8.77015828355848,-10.1019213543007,-0.719973041704905));
#97771=CARTESIAN_POINT('Ctrl Pts',(8.75299937723619,-9.93349546234244,-0.835351913469143));
#97772=CARTESIAN_POINT('Ctrl Pts',(8.72871516126698,-9.5640376440529,-0.988544335314129));
#97773=CARTESIAN_POINT('Ctrl Pts',(8.72195505606398,-9.36297374125027,-1.026338439606));
#97774=CARTESIAN_POINT('Ctrl Pts',(8.72195505606398,-9.17423561284,-1.026338439606));
#97775=CARTESIAN_POINT('Ctrl Pts',(8.72195505606398,-8.98549748442973,-1.026338439606));
#97776=CARTESIAN_POINT('Ctrl Pts',(8.72871516126698,-8.7844335816271,-0.988544335314129));
#97777=CARTESIAN_POINT('Ctrl Pts',(8.75299937723619,-8.41497576333756,-0.835351913469142));
#97778=CARTESIAN_POINT('Ctrl Pts',(8.77015828355848,-8.24654987137926,-0.719973041704905));
#97779=CARTESIAN_POINT('Ctrl Pts',(8.80226283219622,-7.98060481275496,-0.4540279830806));
#97780=CARTESIAN_POINT('Ctrl Pts',(8.81931354586398,-7.86522295898186,-0.285600460274688));
#97781=CARTESIAN_POINT('Ctrl Pts',(8.84334932535928,-7.71202837241176,0.083862965815867));
#97782=CARTESIAN_POINT('Ctrl Pts',(8.85,-7.67423561284,0.284928828397001));
#97783=CARTESIAN_POINT('Ctrl Pts',(8.85,-7.67423561284,0.662394292391));
#97784=CARTESIAN_POINT('Ctrl Pts',(8.84334932535928,-7.71202837241176,0.863460154972134));
#97785=CARTESIAN_POINT('Ctrl Pts',(8.81931354586398,-7.86522295898186,1.23292358106269));
#97786=CARTESIAN_POINT('Ctrl Pts',(8.80226283219622,-7.98060481275496,1.4013511038686));
#97787=CARTESIAN_POINT('Ctrl Pts',(8.77015828355848,-8.24654987137926,1.66729616249291));
#97788=CARTESIAN_POINT('Ctrl Pts',(8.75299937723619,-8.41497576333756,1.78267503425714));
#97789=CARTESIAN_POINT('Ctrl Pts',(8.72871516126698,-8.78443358162711,1.93586745610213));
#97790=CARTESIAN_POINT('Ctrl Pts',(8.72195505606398,-8.98549748442973,1.973661560394));
#97791=CARTESIAN_POINT('Ctrl Pts',(8.72195505606398,-9.36297374125027,1.973661560394));
#97792=CARTESIAN_POINT('Ctrl Pts',(8.72871516126698,-9.5640376440529,1.93586745610213));
#97793=CARTESIAN_POINT('Ctrl Pts',(8.75299937723619,-9.93349546234245,1.78267503425714));
#97794=CARTESIAN_POINT('Ctrl Pts',(8.77015828355847,-10.1019213543007,1.6672961624929));
#97795=CARTESIAN_POINT('Ctrl Pts',(8.78621078736448,-10.2348957846198,1.53432173217382));
#97796=CARTESIAN_POINT('Origin',(4.,-9.92423561284,10.9094726032));
#97797=CARTESIAN_POINT('',(6.61089801788,-9.92423561284,-5.41008957278));
#97798=CARTESIAN_POINT('',(8.47467596136,-9.92423561284,-2.07631242966));
#97799=CARTESIAN_POINT('Origin',(0.,-9.92423561284,0.473661560394));
#97800=CARTESIAN_POINT('',(6.61089801788,-9.92423561284,-2.07631242966));
#97801=CARTESIAN_POINT('',(7.54278698962,-9.92423561284,-2.07631242966));
#97802=CARTESIAN_POINT('',(6.61089801788,-9.92423561284,-3.74320100122));
#97803=CARTESIAN_POINT('Origin',(9.7,-9.17423561284,-2.07631242966));
#97804=CARTESIAN_POINT('',(8.47467596136,-10.2242096029,-2.07631242966));
#97805=CARTESIAN_POINT('',(8.47467596136,-9.81495241206,-2.07631242966));
#97806=CARTESIAN_POINT('',(6.61089801788,-10.2242096029,-2.07631242966));
#97807=CARTESIAN_POINT('',(7.23999999989,-10.2242096029,-2.07631242966));
#97808=CARTESIAN_POINT('',(6.61089801788,-10.0742226079,-2.07631242966));
#97809=CARTESIAN_POINT('Origin',(7.23999999989,-10.2242096029,0.473661560394));
#97810=CARTESIAN_POINT('',(8.81816307332978,-12.6613939105328,-0.276338439790844));
#97811=CARTESIAN_POINT('Ctrl Pts',(8.81816307399792,-12.6613939105698,-0.276338439859058));
#97812=CARTESIAN_POINT('Ctrl Pts',(8.81159014191855,-12.6376118819527,-0.353620022433216));
#97813=CARTESIAN_POINT('Ctrl Pts',(8.80407126472156,-12.6100918009648,-0.429935532759619));
#97814=CARTESIAN_POINT('Ctrl Pts',(8.76084293562039,-12.4486247941201,-0.818571700939171));
#97815=CARTESIAN_POINT('Ctrl Pts',(8.71126631028426,-12.2526596929331,-1.10409615000023));
#97816=CARTESIAN_POINT('Ctrl Pts',(8.61746290023769,-11.8019105710455,-1.55484527188781));
#97817=CARTESIAN_POINT('Ctrl Pts',(8.56695493619419,-11.516409326613,-1.75076635383017));
#97818=CARTESIAN_POINT('Ctrl Pts',(8.49497179593289,-10.8887452246525,-2.01154492600502));
#97819=CARTESIAN_POINT('Ctrl Pts',(8.47467596136091,-10.5464102971449,-2.076312429656));
#97820=CARTESIAN_POINT('Ctrl Pts',(8.47467596136091,-10.2242096029,-2.076312429656));
#97821=CARTESIAN_POINT('',(6.61089801788,-12.6613939106,-0.276338439606));
#97822=CARTESIAN_POINT('',(7.71453053854,-12.6613939106,-0.276338439606));
#97823=CARTESIAN_POINT('Origin',(6.61089801788,-10.2242096029,0.473661560394));
#97824=CARTESIAN_POINT('Origin',(4.,-11.2955559564,-0.276338439606));
#97825=CARTESIAN_POINT('',(8.81816307402,-14.9244482822,-0.276338439606));
#97826=CARTESIAN_POINT('',(6.61089801788,-14.9244482822,-0.276338439606));
#97827=CARTESIAN_POINT('',(7.71453054595,-14.9244482822,-0.276338439606));
#97828=CARTESIAN_POINT('',(6.61089801788,-13.7929210964,-0.276338439606));
#97829=CARTESIAN_POINT('',(8.81816307402,-9.81495241206,-0.276338439606));
#97830=CARTESIAN_POINT('Origin',(4.,-2.81495241206,1.22366156039));
#97831=CARTESIAN_POINT('',(8.81816307334515,-12.6613939101212,1.22366156090261));
#97832=CARTESIAN_POINT('',(8.81816307402,-14.9244482822,1.22366156039));
#97833=CARTESIAN_POINT('',(8.81816307402,-9.81495241206,1.22366156039));
#97834=CARTESIAN_POINT('',(6.61089801788,-12.6613939106,1.22366156039));
#97835=CARTESIAN_POINT('',(7.23999999989,-12.6613939106,1.22366156039));
#97836=CARTESIAN_POINT('',(6.61089801788,-14.9244482822,1.22366156039));
#97837=CARTESIAN_POINT('',(6.61089801788,-13.7929210964,1.22366156039));
#97838=CARTESIAN_POINT('',(7.71453054595,-14.9244482822,1.22366156039));
#97839=CARTESIAN_POINT('Origin',(7.23999999989,-10.2242096029,0.473661560394));
#97840=CARTESIAN_POINT('',(8.47467596136,-10.2242096029,3.02363555044));
#97841=CARTESIAN_POINT('Ctrl Pts',(8.47467596136091,-10.2242096029,3.023635550444));
#97842=CARTESIAN_POINT('Ctrl Pts',(8.47467596136091,-10.5464102971449,3.023635550444));
#97843=CARTESIAN_POINT('Ctrl Pts',(8.49497179593289,-10.8887452246525,2.95886804679302));
#97844=CARTESIAN_POINT('Ctrl Pts',(8.56695493619419,-11.516409326613,2.69808947461818));
#97845=CARTESIAN_POINT('Ctrl Pts',(8.61746290023769,-11.8019105710455,2.50216839267581));
#97846=CARTESIAN_POINT('Ctrl Pts',(8.71126631028426,-12.2526596929331,2.05141927078824));
#97847=CARTESIAN_POINT('Ctrl Pts',(8.76084293562039,-12.4486247941201,1.76589482172717));
#97848=CARTESIAN_POINT('Ctrl Pts',(8.80407126470694,-12.6100918009102,1.37725865367903));
#97849=CARTESIAN_POINT('Ctrl Pts',(8.81159014189213,-12.637611881856,1.30094314348955));
#97850=CARTESIAN_POINT('Ctrl Pts',(8.81816307396325,-12.6613939104444,1.22366156105464));
#97851=CARTESIAN_POINT('',(6.61089801788,-10.2242096029,3.02363555044));
#97852=CARTESIAN_POINT('',(7.54278698962,-10.2242096029,3.02363555044));
#97853=CARTESIAN_POINT('Origin',(6.61089801788,-10.2242096029,0.473661560394));
#97854=CARTESIAN_POINT('Origin',(9.7,-9.17423561284,3.02363555044));
#97855=CARTESIAN_POINT('',(6.61089801788,-9.92423561284,3.02363555044));
#97856=CARTESIAN_POINT('',(6.61089801788,-10.0742226079,3.02363555044));
#97857=CARTESIAN_POINT('',(8.47467596136,-9.92423561284,3.02363555044));
#97858=CARTESIAN_POINT('',(8.47467596136,-9.81495241206,3.02363555044));
#97859=CARTESIAN_POINT('',(7.54278698962,-9.92423561284,3.02363555044));
#97860=CARTESIAN_POINT('Origin',(4.,-9.92423561284,10.9094726032));
#97861=CARTESIAN_POINT('',(6.61089801788,-9.92423561284,6.35741269357));
#97862=CARTESIAN_POINT('Origin',(0.,-9.92423561284,0.473661560394));
#97863=CARTESIAN_POINT('',(6.61089801788,-9.92423561284,4.69052412201));
#97864=CARTESIAN_POINT('Origin',(4.,-8.42423561284,10.9094726032));
#97865=CARTESIAN_POINT('',(6.61089801788,-8.42423561284,6.35741269357));
#97866=CARTESIAN_POINT('',(6.61089801788,-8.42423561284,2.91087308178));
#97867=CARTESIAN_POINT('',(6.61089801788,-8.42423561284,4.63414288768));
#97868=CARTESIAN_POINT('',(8.50779054749,-8.42423561284,2.91087308178));
#97869=CARTESIAN_POINT('Origin',(0.,-8.42423561284,0.473661560394));
#97870=CARTESIAN_POINT('',(7.85,-8.42423561284,2.91087308178));
#97871=CARTESIAN_POINT('Origin',(7.85,-9.17423561284,0.473661560394));
#97872=CARTESIAN_POINT('',(8.81816307402,-6.73702409145,1.22366156039));
#97873=CARTESIAN_POINT('Ctrl Pts',(8.50779054749244,-8.42423561283885,2.91087308178444));
#97874=CARTESIAN_POINT('Ctrl Pts',(8.5146039575556,-8.34694619186358,2.88708890662246));
#97875=CARTESIAN_POINT('Ctrl Pts',(8.52238203382321,-8.27062509791643,2.85956663804855));
#97876=CARTESIAN_POINT('Ctrl Pts',(8.5669490755189,-7.88202266221689,2.69811213638263));
#97877=CARTESIAN_POINT('Ctrl Pts',(8.61745809932542,-7.59651853184558,2.50218906345097));
#97878=CARTESIAN_POINT('Ctrl Pts',(8.71126345553147,-7.14576485501596,2.05143538662135));
#97879=CARTESIAN_POINT('Ctrl Pts',(8.76084110174091,-6.94979776054387,1.76590805043681));
#97880=CARTESIAN_POINT('Ctrl Pts',(8.80407059609279,-6.78832806722086,1.3772654408237));
#97881=CARTESIAN_POINT('Ctrl Pts',(8.81158985094324,-6.76080690738419,1.30094656440485));
#97882=CARTESIAN_POINT('Ctrl Pts',(8.81816307401973,-6.73702409144815,1.22366156039055));
#97883=CARTESIAN_POINT('',(6.61089801788,-6.73702409145,1.22366156039));
#97884=CARTESIAN_POINT('',(7.71453054595,-6.73702409145,1.22366156039));
#97885=CARTESIAN_POINT('Origin',(6.61089801788,-9.17423561284,0.473661560394));
#97886=CARTESIAN_POINT('Origin',(4.,-2.81495241206,1.22366156039));
#97887=CARTESIAN_POINT('',(8.81816307402,-5.78170707891,1.22366156039));
#97888=CARTESIAN_POINT('',(8.81816307402,-9.81495241206,1.22366156039));
#97889=CARTESIAN_POINT('',(6.61089801788,-5.78170707891,1.22366156039));
#97890=CARTESIAN_POINT('',(7.71453054595,-5.78170707891,1.22366156039));
#97891=CARTESIAN_POINT('',(6.61089801788,-6.25936558518,1.22366156039));
#97892=CARTESIAN_POINT('Origin',(4.,-8.42423561284,10.9094726032));
#97893=CARTESIAN_POINT('',(6.61089801788,-8.42423561284,-1.963549961));
#97894=CARTESIAN_POINT('',(6.61089801788,-8.42423561284,-5.41008957278));
#97895=CARTESIAN_POINT('',(6.61089801788,-8.42423561284,-3.68681976689));
#97896=CARTESIAN_POINT('',(8.50779054749,-8.42423561284,-1.963549961));
#97897=CARTESIAN_POINT('',(7.85,-8.42423561284,-1.963549961));
#97898=CARTESIAN_POINT('Origin',(0.,-8.42423561284,0.473661560394));
#97899=CARTESIAN_POINT('Origin',(7.85,-9.17423561284,0.473661560394));
#97900=CARTESIAN_POINT('',(8.81816307402,-6.73702409145,-0.276338439606));
#97901=CARTESIAN_POINT('',(6.61089801788,-6.73702409145,-0.276338439606));
#97902=CARTESIAN_POINT('',(7.71453054595,-6.73702409145,-0.276338439606));
#97903=CARTESIAN_POINT('Ctrl Pts',(8.50779054749224,-8.42423561284108,-1.96354996099712));
#97904=CARTESIAN_POINT('Ctrl Pts',(8.51460395755545,-8.34694619186505,-1.93976578583499));
#97905=CARTESIAN_POINT('Ctrl Pts',(8.52238203382313,-8.27062509791715,-1.91224351726085));
#97906=CARTESIAN_POINT('Ctrl Pts',(8.5669490755189,-7.88202266221689,-1.75078901559463));
#97907=CARTESIAN_POINT('Ctrl Pts',(8.61745809932542,-7.59651853184558,-1.55486594266297));
#97908=CARTESIAN_POINT('Ctrl Pts',(8.71126345553147,-7.14576485501596,-1.10411226583335));
#97909=CARTESIAN_POINT('Ctrl Pts',(8.76084110174091,-6.94979776054387,-0.818584929648813));
#97910=CARTESIAN_POINT('Ctrl Pts',(8.80407059609266,-6.78832806722135,-0.429942320036871));
#97911=CARTESIAN_POINT('Ctrl Pts',(8.811589850943,-6.76080690738505,-0.353623443619237));
#97912=CARTESIAN_POINT('Ctrl Pts',(8.81816307401943,-6.73702409144926,-0.276338439606177));
#97913=CARTESIAN_POINT('Origin',(6.61089801788,-9.17423561284,0.473661560394));
#97914=CARTESIAN_POINT('Origin',(4.,-11.2955559564,-0.276338439606));
#97915=CARTESIAN_POINT('',(6.61089801788,-5.78170707891,-0.276338439606));
#97916=CARTESIAN_POINT('',(6.61089801788,-6.25936558518,-0.276338439606));
#97917=CARTESIAN_POINT('',(8.81816307402,-5.78170707891,-0.276338439606));
#97918=CARTESIAN_POINT('',(7.71453054595,-5.78170707891,-0.276338439606));
#97919=CARTESIAN_POINT('',(8.81816307402,-9.81495241206,-0.276338439606));
#97920=CARTESIAN_POINT('Origin',(-4.8,-19.0742356128,-2.12633843961));
#97921=CARTESIAN_POINT('',(-4.8,-19.3742356128,-5.5013690143));
#97922=CARTESIAN_POINT('Origin',(-4.8,-19.0742356128,-5.5013690143));
#97923=CARTESIAN_POINT('',(-4.8,-19.3742356128,6.1986309857));
#97924=CARTESIAN_POINT('Origin',(-4.8,-19.0742356128,6.1986309857));
#97925=CARTESIAN_POINT('',(-4.8,-19.3742356128,0.348630985699));
#97926=CARTESIAN_POINT('Origin',(0.,-19.3742356128,0.473661560394));
#97927=CARTESIAN_POINT('',(-8.4371184738,-19.3742356128,6.46845362177));
#97928=CARTESIAN_POINT('',(-10.7402266336,-19.3742356128,6.46845362177));
#97929=CARTESIAN_POINT('',(-9.58867255369,-19.3742356128,6.46845362177));
#97930=CARTESIAN_POINT('',(-6.81380166599,-19.3742356128,-9.7665584986));
#97931=CARTESIAN_POINT('Origin',(0.,-19.3742356128,0.473661560394));
#97932=CARTESIAN_POINT('',(-6.67999195052,-19.3742356128,-10.0163199635));
#97933=CARTESIAN_POINT('Origin',(-6.97999195052,-19.3742356128,-10.0163199635));
#97934=CARTESIAN_POINT('',(-6.67999195052,-19.3742356128,-13.3776272862));
#97935=CARTESIAN_POINT('',(-6.67999195052,-19.3742356128,-11.6969736248));
#97936=CARTESIAN_POINT('',(-6.5054999889,-19.3742356128,-13.6501116569));
#97937=CARTESIAN_POINT('Origin',(-6.37999195052,-19.3742356128,-13.3776272862));
#97938=CARTESIAN_POINT('',(-5.2992520131,-19.3742356128,-14.1455185843));
#97939=CARTESIAN_POINT('Origin',(0.,-19.3742356128,0.473661560394));
#97940=CARTESIAN_POINT('',(-4.92636192076,-19.3742356128,-13.9928850408));
#97941=CARTESIAN_POINT('Origin',(-5.19701563986,-19.3742356128,-13.8634765236));
#97942=CARTESIAN_POINT('',(-4.56454191842,-19.3742356128,-13.8364811917));
#97943=CARTESIAN_POINT('Origin',(-4.65570820166,-19.3742356128,-14.1222935581));
#97944=CARTESIAN_POINT('',(-3.37623759365,-19.3742356128,-14.1624666237));
#97945=CARTESIAN_POINT('Origin',(0.,-19.3742356128,0.473661560394));
#97946=CARTESIAN_POINT('',(-3.1436702163,-19.3742356128,-14.4547898034));
#97947=CARTESIAN_POINT('Origin',(-3.4436702163,-19.3742356128,-14.4547898034));
#97948=CARTESIAN_POINT('',(-3.1436702163,-19.3742356128,-14.5088629165));
#97949=CARTESIAN_POINT('',(-3.1436702163,-19.3742356128,-14.48182636));
#97950=CARTESIAN_POINT('',(-2.89961126973,-19.3742356128,-14.8036011029));
#97951=CARTESIAN_POINT('Origin',(-2.8436702163,-19.3742356128,-14.5088629165));
#97952=CARTESIAN_POINT('',(2.89961126973,-19.3742356128,-14.8036011029));
#97953=CARTESIAN_POINT('Origin',(0.,-19.3742356128,0.473661560394));
#97954=CARTESIAN_POINT('',(3.1436702163,-19.3742356128,-14.5088629165));
#97955=CARTESIAN_POINT('Origin',(2.8436702163,-19.3742356128,-14.5088629165));
#97956=CARTESIAN_POINT('',(3.1436702163,-19.3742356128,-14.4547898034));
#97957=CARTESIAN_POINT('',(3.1436702163,-19.3742356128,-14.48182636));
#97958=CARTESIAN_POINT('',(3.37623759365,-19.3742356128,-14.1624666237));
#97959=CARTESIAN_POINT('Origin',(3.4436702163,-19.3742356128,-14.4547898034));
#97960=CARTESIAN_POINT('',(4.62312919377,-19.3742356128,-13.8176611554));
#97961=CARTESIAN_POINT('Origin',(0.,-19.3742356128,0.473661560394));
#97962=CARTESIAN_POINT('',(4.98558691274,-19.3742356128,-13.9725813932));
#97963=CARTESIAN_POINT('Origin',(4.71546562382,-19.3742356128,-14.1030976346));
#97964=CARTESIAN_POINT('',(5.35909918268,-19.3742356128,-14.1236860052));
#97965=CARTESIAN_POINT('Origin',(5.25570820166,-19.3742356128,-13.8420651518));
#97966=CARTESIAN_POINT('',(6.5054999889,-19.3742356128,-13.6501116569));
#97967=CARTESIAN_POINT('Origin',(0.,-19.3742356128,0.473661560394));
#97968=CARTESIAN_POINT('',(6.67999195052,-19.3742356128,-13.3776272862));
#97969=CARTESIAN_POINT('Origin',(6.37999195052,-19.3742356128,-13.3776272862));
#97970=CARTESIAN_POINT('',(6.67999195052,-19.3742356128,-10.0163199635));
#97971=CARTESIAN_POINT('',(6.67999195052,-19.3742356128,-11.6969736248));
#97972=CARTESIAN_POINT('',(6.81380166599,-19.3742356128,-9.7665584986));
#97973=CARTESIAN_POINT('Origin',(6.97999195052,-19.3742356128,-10.0163199635));
#97974=CARTESIAN_POINT('',(10.7402266336,-19.3742356128,6.46845362177));
#97975=CARTESIAN_POINT('Origin',(0.,-19.3742356128,0.473661560394));
#97976=CARTESIAN_POINT('',(8.4371184738,-19.3742356128,6.46845362177));
#97977=CARTESIAN_POINT('',(9.58867255369,-19.3742356128,6.46845362177));
#97978=CARTESIAN_POINT('Origin',(0.,-19.3742356128,0.473661560394));
#97979=CARTESIAN_POINT('Origin',(-4.2,-19.3742356128,-5.5013690143));
#97980=CARTESIAN_POINT('',(-4.2,-19.3742356128,6.7986309857));
#97981=CARTESIAN_POINT('Origin',(-4.2,-19.3742356128,6.1986309857));
#97982=CARTESIAN_POINT('',(4.2,-19.3742356128,6.7986309857));
#97983=CARTESIAN_POINT('',(0.,-19.3742356128,6.7986309857));
#97984=CARTESIAN_POINT('',(4.8,-19.3742356128,6.1986309857));
#97985=CARTESIAN_POINT('Origin',(4.2,-19.3742356128,6.1986309857));
#97986=CARTESIAN_POINT('',(4.8,-19.3742356128,-5.5013690143));
#97987=CARTESIAN_POINT('',(4.8,-19.3742356128,-2.12633843961));
#97988=CARTESIAN_POINT('Origin',(4.2,-19.3742356128,-5.5013690143));
#97989=CARTESIAN_POINT('Origin',(0.,-18.0242356128,0.473661560394));
#97990=CARTESIAN_POINT('',(-6.81380166599,-16.6742356128,-9.7665584986));
#97991=CARTESIAN_POINT('',(-6.81380166599,-18.0242356128,-9.7665584986));
#97992=CARTESIAN_POINT('',(-10.7402266336,-16.6742356128,6.46845362177));
#97993=CARTESIAN_POINT('',(-10.7402266336,-18.0242356128,6.46845362177));
#97994=CARTESIAN_POINT('Origin',(0.,-16.6742356128,0.473661560394));
#97995=CARTESIAN_POINT('Origin',(10.7402266336,-19.3742356128,6.46845362177));
#97996=CARTESIAN_POINT('',(-8.4371184738,-16.6742356128,6.46845362177));
#97997=CARTESIAN_POINT('',(-8.4371184738,-18.0242356128,6.46845362177));
#97998=CARTESIAN_POINT('',(-9.58867255369,-16.6742356128,6.46845362177));
#97999=CARTESIAN_POINT('Origin',(0.,-18.0242356128,0.473661560394));
#98000=CARTESIAN_POINT('',(8.4371184738,-16.6742356128,6.46845362177));
#98001=CARTESIAN_POINT('Origin',(0.,-16.6742356128,0.473661560394));
#98002=CARTESIAN_POINT('',(8.4371184738,-18.0242356128,6.46845362177));
#98003=CARTESIAN_POINT('Origin',(10.7402266336,-19.3742356128,6.46845362177));
#98004=CARTESIAN_POINT('',(10.7402266336,-16.6742356128,6.46845362177));
#98005=CARTESIAN_POINT('',(10.7402266336,-18.0242356128,6.46845362177));
#98006=CARTESIAN_POINT('',(9.58867255369,-16.6742356128,6.46845362177));
#98007=CARTESIAN_POINT('Origin',(0.,-18.0242356128,0.473661560394));
#98008=CARTESIAN_POINT('',(6.81380166599,-16.6742356128,-9.7665584986));
#98009=CARTESIAN_POINT('',(6.81380166599,-18.0242356128,-9.7665584986));
#98010=CARTESIAN_POINT('Origin',(0.,-16.6742356128,0.473661560394));
#98011=CARTESIAN_POINT('Origin',(6.97999195052,-18.0242356128,-10.0163199635));
#98012=CARTESIAN_POINT('',(6.67999195052,-16.6742356128,-10.0163199635));
#98013=CARTESIAN_POINT('',(6.67999195052,-18.0242356128,-10.0163199635));
#98014=CARTESIAN_POINT('Origin',(6.97999195052,-16.6742356128,-10.0163199635));
#98015=CARTESIAN_POINT('Origin',(6.67999195052,-19.3742356128,-9.85434442048));
#98016=CARTESIAN_POINT('',(6.67999195052,-16.6742356128,-13.3776272862));
#98017=CARTESIAN_POINT('',(6.67999195052,-18.0242356128,-13.3776272862));
#98018=CARTESIAN_POINT('',(6.67999195052,-16.6742356128,-11.6969736248));
#98019=CARTESIAN_POINT('Origin',(6.37999195052,-18.0242356128,-13.3776272862));
#98020=CARTESIAN_POINT('',(6.5054999889,-16.6742356128,-13.6501116569));
#98021=CARTESIAN_POINT('Origin',(6.37999195052,-16.6742356128,-13.3776272862));
#98022=CARTESIAN_POINT('',(6.5054999889,-18.0242356128,-13.6501116569));
#98023=CARTESIAN_POINT('Origin',(0.,-18.0242356128,0.473661560394));
#98024=CARTESIAN_POINT('',(5.35909918268,-16.6742356128,-14.1236860052));
#98025=CARTESIAN_POINT('Origin',(0.,-16.6742356128,0.473661560394));
#98026=CARTESIAN_POINT('',(5.35909918268,-18.0242356128,-14.1236860052));
#98027=CARTESIAN_POINT('Origin',(5.25570820166,-18.0242356128,-13.8420651518));
#98028=CARTESIAN_POINT('',(4.98558691274,-16.6742356128,-13.9725813932));
#98029=CARTESIAN_POINT('Origin',(5.25570820166,-16.6742356128,-13.8420651518));
#98030=CARTESIAN_POINT('',(4.98558691274,-18.0242356128,-13.9725813932));
#98031=CARTESIAN_POINT('Origin',(4.71546562382,-18.0242356128,-14.1030976346));
#98032=CARTESIAN_POINT('',(4.62312919377,-16.6742356128,-13.8176611554));
#98033=CARTESIAN_POINT('',(4.62312919377,-18.0242356128,-13.8176611554));
#98034=CARTESIAN_POINT('Origin',(4.71546562382,-16.6742356128,-14.1030976346));
#98035=CARTESIAN_POINT('Origin',(0.,-18.0242356128,0.473661560394));
#98036=CARTESIAN_POINT('',(3.37623759365,-16.6742356128,-14.1624666237));
#98037=CARTESIAN_POINT('',(3.37623759365,-18.0242356128,-14.1624666237));
#98038=CARTESIAN_POINT('Origin',(0.,-16.6742356128,0.473661560394));
#98039=CARTESIAN_POINT('Origin',(3.4436702163,-18.0242356128,-14.4547898034));
#98040=CARTESIAN_POINT('',(3.1436702163,-16.6742356128,-14.4547898034));
#98041=CARTESIAN_POINT('',(3.1436702163,-18.0242356128,-14.4547898034));
#98042=CARTESIAN_POINT('Origin',(3.4436702163,-16.6742356128,-14.4547898034));
#98043=CARTESIAN_POINT('Origin',(3.1436702163,-19.3742356128,-14.2141757917));
#98044=CARTESIAN_POINT('',(3.1436702163,-16.6742356128,-14.5088629165));
#98045=CARTESIAN_POINT('',(3.1436702163,-16.6742356128,-14.48182636));
#98046=CARTESIAN_POINT('',(3.1436702163,-18.0242356128,-14.5088629165));
#98047=CARTESIAN_POINT('Origin',(2.8436702163,-18.0242356128,-14.5088629165));
#98048=CARTESIAN_POINT('',(2.89961126973,-16.6742356128,-14.8036011029));
#98049=CARTESIAN_POINT('Origin',(2.8436702163,-16.6742356128,-14.5088629165));
#98050=CARTESIAN_POINT('',(2.89961126973,-18.0242356128,-14.8036011029));
#98051=CARTESIAN_POINT('Origin',(0.,-18.0242356128,0.473661560394));
#98052=CARTESIAN_POINT('',(-2.89961126973,-16.6742356128,-14.8036011029));
#98053=CARTESIAN_POINT('',(-2.89961126973,-18.0242356128,-14.8036011029));
#98054=CARTESIAN_POINT('Origin',(0.,-16.6742356128,0.473661560394));
#98055=CARTESIAN_POINT('Origin',(-2.8436702163,-18.0242356128,-14.5088629165));
#98056=CARTESIAN_POINT('',(-3.1436702163,-16.6742356128,-14.5088629165));
#98057=CARTESIAN_POINT('Origin',(-2.8436702163,-16.6742356128,-14.5088629165));
#98058=CARTESIAN_POINT('',(-3.1436702163,-18.0242356128,-14.5088629165));
#98059=CARTESIAN_POINT('Origin',(-3.1436702163,-19.3742356128,-14.2141757917));
#98060=CARTESIAN_POINT('',(-3.1436702163,-16.6742356128,-14.4547898034));
#98061=CARTESIAN_POINT('',(-3.1436702163,-18.0242356128,-14.4547898034));
#98062=CARTESIAN_POINT('',(-3.1436702163,-16.6742356128,-14.48182636));
#98063=CARTESIAN_POINT('Origin',(-3.4436702163,-18.0242356128,-14.4547898034));
#98064=CARTESIAN_POINT('',(-3.37623759365,-16.6742356128,-14.1624666237));
#98065=CARTESIAN_POINT('',(-3.37623759365,-18.0242356128,-14.1624666237));
#98066=CARTESIAN_POINT('Origin',(-3.4436702163,-16.6742356128,-14.4547898034));
#98067=CARTESIAN_POINT('Origin',(0.,-18.0242356128,0.473661560394));
#98068=CARTESIAN_POINT('',(-4.56454191842,-16.6742356128,-13.8364811917));
#98069=CARTESIAN_POINT('',(-4.56454191842,-18.0242356128,-13.8364811917));
#98070=CARTESIAN_POINT('Origin',(0.,-16.6742356128,0.473661560394));
#98071=CARTESIAN_POINT('Origin',(-4.65570820166,-18.0242356128,-14.1222935581));
#98072=CARTESIAN_POINT('',(-4.92636192076,-16.6742356128,-13.9928850408));
#98073=CARTESIAN_POINT('',(-4.92636192076,-18.0242356128,-13.9928850408));
#98074=CARTESIAN_POINT('Origin',(-4.65570820166,-16.6742356128,-14.1222935581));
#98075=CARTESIAN_POINT('Origin',(-5.19701563986,-18.0242356128,-13.8634765236));
#98076=CARTESIAN_POINT('',(-5.2992520131,-16.6742356128,-14.1455185843));
#98077=CARTESIAN_POINT('Origin',(-5.19701563986,-16.6742356128,-13.8634765236));
#98078=CARTESIAN_POINT('',(-5.2992520131,-18.0242356128,-14.1455185843));
#98079=CARTESIAN_POINT('Origin',(0.,-18.0242356128,0.473661560394));
#98080=CARTESIAN_POINT('',(-6.5054999889,-16.6742356128,-13.6501116569));
#98081=CARTESIAN_POINT('',(-6.5054999889,-18.0242356128,-13.6501116569));
#98082=CARTESIAN_POINT('Origin',(0.,-16.6742356128,0.473661560394));
#98083=CARTESIAN_POINT('Origin',(-6.37999195052,-18.0242356128,-13.3776272862));
#98084=CARTESIAN_POINT('',(-6.67999195052,-16.6742356128,-13.3776272862));
#98085=CARTESIAN_POINT('Origin',(-6.37999195052,-16.6742356128,-13.3776272862));
#98086=CARTESIAN_POINT('',(-6.67999195052,-18.0242356128,-13.3776272862));
#98087=CARTESIAN_POINT('Origin',(-6.67999195052,-19.3742356128,-9.85434442048));
#98088=CARTESIAN_POINT('',(-6.67999195052,-16.6742356128,-10.0163199635));
#98089=CARTESIAN_POINT('',(-6.67999195052,-18.0242356128,-10.0163199635));
#98090=CARTESIAN_POINT('',(-6.67999195052,-16.6742356128,-11.6969736248));
#98091=CARTESIAN_POINT('Origin',(-6.97999195052,-18.0242356128,-10.0163199635));
#98092=CARTESIAN_POINT('Origin',(-6.97999195052,-16.6742356128,-10.0163199635));
#98093=CARTESIAN_POINT('Origin',(6.61089801788,-5.78170707891,0.473661560394));
#98094=CARTESIAN_POINT('',(6.61089801788,-5.78170707891,6.35741269357));
#98095=CARTESIAN_POINT('Origin',(0.,-5.78170707891,0.473661560394));
#98096=CARTESIAN_POINT('',(6.61089801788,-5.78170707891,3.79053712698));
#98097=CARTESIAN_POINT('Origin',(6.61089801788,-14.9244482822,0.473661560394));
#98098=CARTESIAN_POINT('',(6.61089801788,-12.0242356128,6.35741269357));
#98099=CARTESIAN_POINT('Origin',(6.61089801788,-14.9244482822,0.473661560394));
#98100=CARTESIAN_POINT('',(6.61089801788,-14.9244482822,6.35741269357));
#98101=CARTESIAN_POINT('',(6.61089801788,-12.0242356128,6.35741269357));
#98102=CARTESIAN_POINT('',(6.61089801788,-14.9244482822,3.79053712698));
#98103=CARTESIAN_POINT('Origin',(13.7258691788,-14.9244482822,0.473661560394));
#98104=CARTESIAN_POINT('Origin',(0.,-14.9244482822,0.473661560394));
#98105=CARTESIAN_POINT('Origin',(13.7258691788,-14.9244482822,0.473661560394));
#98106=CARTESIAN_POINT('',(6.61089801788,-14.9244482822,-5.41008957278));
#98107=CARTESIAN_POINT('Origin',(0.,-14.9244482822,0.473661560394));
#98108=CARTESIAN_POINT('',(6.61089801788,-14.9244482822,-2.84321400619));
#98109=CARTESIAN_POINT('Origin',(6.61089801788,-14.9244482822,0.473661560394));
#98110=CARTESIAN_POINT('',(6.61089801788,-12.0242356128,-5.41008957278));
#98111=CARTESIAN_POINT('Origin',(0.,-9.81495241206,0.473661560394));
#98112=CARTESIAN_POINT('',(-8.40228522294909E-15,-16.6742356128,9.323661560394));
#98113=CARTESIAN_POINT('',(-8.40228522294909E-15,-9.81495241206,9.323661560394));
#98114=CARTESIAN_POINT('Origin',(0.,-16.6742356128,0.473661560394));
#98115=CARTESIAN_POINT('',(6.61089801788,-5.78170707891,-5.41008957278));
#98116=CARTESIAN_POINT('Origin',(0.,-5.78170707891,0.473661560394));
#98117=CARTESIAN_POINT('',(6.61089801788,-12.0242356128,-5.41008957278));
#98118=CARTESIAN_POINT('Origin',(6.61089801788,-14.9244482822,0.473661560394));
#98119=CARTESIAN_POINT('',(6.61089801788,-5.78170707891,-2.84321400619));
#98120=CARTESIAN_POINT('Origin',(6.61089801788,-5.78170707891,0.473661560394));
#98121=CARTESIAN_POINT('Origin',(-4.2,-19.0742356128,6.1986309857));
#98122=CARTESIAN_POINT('',(-4.2,-19.0742356128,6.4986309857));
#98123=CARTESIAN_POINT('Origin',(-4.2,-19.0742356128,6.1986309857));
#98124=CARTESIAN_POINT('Origin',(-4.2,-19.0742356128,6.7986309857));
#98125=CARTESIAN_POINT('Origin',(-4.2,-13.6742356128,6.1986309857));
#98126=CARTESIAN_POINT('',(-4.2,-11.8742356128,6.4986309857));
#98127=CARTESIAN_POINT('Origin',(0.,-19.0742356128,6.7986309857));
#98128=CARTESIAN_POINT('',(4.2,-19.0742356128,6.4986309857));
#98129=CARTESIAN_POINT('',(-8.881784197E-16,-19.0742356128,6.4986309857));
#98130=CARTESIAN_POINT('Origin',(4.2,-19.0742356128,6.7986309857));
#98131=CARTESIAN_POINT('Origin',(0.,-4.67423561284,6.4986309857));
#98132=CARTESIAN_POINT('',(4.2,-13.6742356128,6.4986309857));
#98133=CARTESIAN_POINT('Origin',(4.2,-19.0742356128,6.1986309857));
#98134=CARTESIAN_POINT('',(4.5,-19.0742356128,6.1986309857));
#98135=CARTESIAN_POINT('Origin',(4.2,-19.0742356128,6.1986309857));
#98136=CARTESIAN_POINT('Origin',(4.8,-19.0742356128,6.1986309857));
#98137=CARTESIAN_POINT('Origin',(4.2,-13.6742356128,6.1986309857));
#98138=CARTESIAN_POINT('',(4.5,-11.8742356128,6.1986309857));
#98139=CARTESIAN_POINT('Origin',(4.8,-19.0742356128,-2.12633843961));
#98140=CARTESIAN_POINT('',(4.5,-19.0742356128,-5.5013690143));
#98141=CARTESIAN_POINT('',(4.5,-19.0742356128,0.348630985699));
#98142=CARTESIAN_POINT('Origin',(4.8,-19.0742356128,-5.5013690143));
#98143=CARTESIAN_POINT('Origin',(4.5,-4.67423561284,6.4986309857));
#98144=CARTESIAN_POINT('',(4.5,-13.6742356128,-5.5013690143));
#98145=CARTESIAN_POINT('Ctrl Pts',(4.20000000308,-18.6809100802,-5.80136900064));
#98146=CARTESIAN_POINT('Ctrl Pts',(4.13201933245,-18.7060691672,-5.80136900054));
#98147=CARTESIAN_POINT('Ctrl Pts',(4.06403866191,-18.7312282542,-5.8232621298));
#98148=CARTESIAN_POINT('Ctrl Pts',(4.00438515095,-18.7533055279,-5.86715848437));
#98149=CARTESIAN_POINT('Ctrl Pts',(3.96107032752,-18.7693359879,-5.92716273862));
#98150=CARTESIAN_POINT('Ctrl Pts',(3.93695198573,-18.7782619879,-5.99493428879));
#98151=CARTESIAN_POINT('Ctrl Pts',(4.21444980228,-18.7589979661,-5.80136893282));
#98152=CARTESIAN_POINT('Ctrl Pts',(4.14870278107,-18.7823836855,-5.80464328508));
#98153=CARTESIAN_POINT('Ctrl Pts',(4.08401026512,-18.8057694048,-5.82817358597));
#98154=CARTESIAN_POINT('Ctrl Pts',(4.02779990888,-18.8265241376,-5.87164554118));
#98155=CARTESIAN_POINT('Ctrl Pts',(3.98697421869,-18.8420998044,-5.92969663234));
#98156=CARTESIAN_POINT('Ctrl Pts',(3.96404157784,-18.8514591938,-5.99493417698));
#98157=CARTESIAN_POINT('Ctrl Pts',(4.22827546583,-18.8373868265,-5.80049863859));
#98158=CARTESIAN_POINT('Ctrl Pts',(4.16490990067,-18.8591197488,-5.8066369302));
#98159=CARTESIAN_POINT('Ctrl Pts',(4.10341065724,-18.8808526711,-5.83146844409));
#98160=CARTESIAN_POINT('Ctrl Pts',(4.0503920793,-18.9003289652,-5.87438626363));
#98161=CARTESIAN_POINT('Ctrl Pts',(4.01183648058,-18.9153528523,-5.93052115145));
#98162=CARTESIAN_POINT('Ctrl Pts',(3.98996106595,-18.9249385271,-5.99330264064));
#98163=CARTESIAN_POINT('Ctrl Pts',(4.24142568441,-18.9160882934,-5.79890830556));
#98164=CARTESIAN_POINT('Ctrl Pts',(4.18051060715,-18.9362628974,-5.80752351469));
#98165=CARTESIAN_POINT('Ctrl Pts',(4.12207728309,-18.9564375015,-5.83336652821));
#98166=CARTESIAN_POINT('Ctrl Pts',(4.07201635859,-18.9746713345,-5.87563301391));
#98167=CARTESIAN_POINT('Ctrl Pts',(4.03553864585,-18.9890689835,-5.92990313712));
#98168=CARTESIAN_POINT('Ctrl Pts',(4.01461432289,-18.9987108858,-5.9903211697));
#98169=CARTESIAN_POINT('Ctrl Pts',(4.2538376014,-18.9950222816,-5.79673916481));
#98170=CARTESIAN_POINT('Ctrl Pts',(4.19537771422,-19.0137178049,-5.80747373633));
#98171=CARTESIAN_POINT('Ctrl Pts',(4.13985677188,-19.0324133281,-5.83407978878));
#98172=CARTESIAN_POINT('Ctrl Pts',(4.09252688404,-19.0494360536,-5.87562478381));
#98173=CARTESIAN_POINT('Ctrl Pts',(4.05794935095,-19.0631474974,-5.92809450339));
#98174=CARTESIAN_POINT('Ctrl Pts',(4.03788343644,-19.0727011908,-5.98625455018));
#98175=CARTESIAN_POINT('Ctrl Pts',(4.26546731361,-19.0742356128,-5.79413860092));
#98176=CARTESIAN_POINT('Ctrl Pts',(4.20941600096,-19.0915169389,-5.80667244675));
#98177=CARTESIAN_POINT('Ctrl Pts',(4.15663577279,-19.1087982649,-5.83383457041));
#98178=CARTESIAN_POINT('Ctrl Pts',(4.11181833689,-19.1246355845,-5.87461401092));
#98179=CARTESIAN_POINT('Ctrl Pts',(4.07897573734,-19.1376111454,-5.92536020439));
#98180=CARTESIAN_POINT('Ctrl Pts',(4.05968611194,-19.146953353,-5.98137917153));
#98181=CARTESIAN_POINT('',(4.26546731361,-19.0742356128,-5.79413860092));
#98182=CARTESIAN_POINT('Origin',(4.33093462721,-19.0742356128,-6.08690818754));
#98183=CARTESIAN_POINT('',(4.20000000673865,-18.6809100779312,-5.80136900746964));
#98184=CARTESIAN_POINT('Ctrl Pts',(4.26546731361,-19.0742356128,-5.79413860092));
#98185=CARTESIAN_POINT('Ctrl Pts',(4.25718116343965,-19.0177962514537,-5.79599149826871));
#98186=CARTESIAN_POINT('Ctrl Pts',(4.24841774144974,-18.9615220782279,-5.79758138057646));
#98187=CARTESIAN_POINT('Ctrl Pts',(4.23921637206803,-18.9054095339776,-5.79879450761291));
#98188=CARTESIAN_POINT('Ctrl Pts',(4.22817173449333,-18.8380562206902,-5.80025065483338));
#98189=CARTESIAN_POINT('Ctrl Pts',(4.21649704322489,-18.7709427807032,-5.80116455660017));
#98190=CARTESIAN_POINT('Ctrl Pts',(4.20426682708576,-18.7040984271016,-5.80133862753531));
#98191=CARTESIAN_POINT('Ctrl Pts',(4.20285195518481,-18.6963654323146,-5.8013587652068));
#98192=CARTESIAN_POINT('Ctrl Pts',(4.201429643321,-18.6886359881787,-5.80136899394372));
#98193=CARTESIAN_POINT('Ctrl Pts',(4.20000000019741,-18.6809100812668,-5.80136900064));
#98194=CARTESIAN_POINT('Origin',(4.20005977102284,-18.680887963059,-6.10146134989777));
#98195=CARTESIAN_POINT('Origin',(4.33093462721,-19.0742356128,-6.08690818754));
#98196=CARTESIAN_POINT('Origin',(4.33093462721,-19.0742356128,-6.08690818754));
#98197=CARTESIAN_POINT('Origin',(4.2,-19.0742356128,-5.5013690143));
#98198=CARTESIAN_POINT('Origin',(4.2,-19.0742356128,-5.5013690143));
#98199=CARTESIAN_POINT('Origin',(4.2,-13.6742356128,-5.5013690143));
#98200=CARTESIAN_POINT('',(4.2,-11.6775728158,-5.8013690143));
#98201=CARTESIAN_POINT('Origin',(-1.50990331349E-14,-20.2352955315,-6.1013690143));
#98202=CARTESIAN_POINT('',(-4.2,-18.6809100188,-5.8013690143));
#98203=CARTESIAN_POINT('Origin',(4.4408920985E-16,-20.2352955315,-5.8013690143));
#98204=CARTESIAN_POINT('Origin',(-4.20006010219018,-18.6808887946701,-6.10146136541638));
#98205=CARTESIAN_POINT('Origin',(0.,-4.67423561284,-5.8013690143));
#98206=CARTESIAN_POINT('',(-4.2,-13.6742356128,-5.8013690143));
#98207=CARTESIAN_POINT('Ctrl Pts',(-4.26546734067,-19.0742356128,-5.79413853556));
#98208=CARTESIAN_POINT('Ctrl Pts',(-4.20941603025,-19.0915169379,-5.80667236858));
#98209=CARTESIAN_POINT('Ctrl Pts',(-4.15663580604,-19.1087982629,-5.83383447647));
#98210=CARTESIAN_POINT('Ctrl Pts',(-4.11181837608,-19.1246355815,-5.87461389924));
#98211=CARTESIAN_POINT('Ctrl Pts',(-4.0789757843,-19.1376111412,-5.92536007425));
#98212=CARTESIAN_POINT('Ctrl Pts',(-4.05968616788,-19.1469533476,-5.98137902326));
#98213=CARTESIAN_POINT('Ctrl Pts',(-4.25383581433,-18.995009694,-5.79673942591));
#98214=CARTESIAN_POINT('Ctrl Pts',(-4.19537554889,-19.0137054404,-5.80747368304));
#98215=CARTESIAN_POINT('Ctrl Pts',(-4.13985417963,-19.0324011868,-5.83407961226));
#98216=CARTESIAN_POINT('Ctrl Pts',(-4.09252390601,-19.0494240988,-5.87562468998));
#98217=CARTESIAN_POINT('Ctrl Pts',(-4.05794611539,-19.0631356574,-5.92809464302));
#98218=CARTESIAN_POINT('Ctrl Pts',(-4.03788009887,-19.0726893818,-5.98625499045));
#98219=CARTESIAN_POINT('Ctrl Pts',(-4.24142181064,-18.9160629516,-5.7989087319));
#98220=CARTESIAN_POINT('Ctrl Pts',(-4.1805059538,-18.9362380267,-5.80752320608));
#98221=CARTESIAN_POINT('Ctrl Pts',(-4.1220717118,-18.9564131018,-5.8333659072));
#98222=CARTESIAN_POINT('Ctrl Pts',(-4.07200993757,-18.9746473194,-5.87563254882));
#98223=CARTESIAN_POINT('Ctrl Pts',(-4.03553165095,-18.9890451839,-5.92990317159));
#98224=CARTESIAN_POINT('Ctrl Pts',(-4.01460709459,-18.9986871093,-5.99032185261));
#98225=CARTESIAN_POINT('Ctrl Pts',(-4.2282770598,-18.8373949885,-5.80049881029));
#98226=CARTESIAN_POINT('Ctrl Pts',(-4.16491182009,-18.8591277431,-5.80663741972));
#98227=CARTESIAN_POINT('Ctrl Pts',(-4.10341297162,-18.8808604976,-5.83146908674));
#98228=CARTESIAN_POINT('Ctrl Pts',(-4.05039476614,-18.9003366584,-5.8743868734));
#98229=CARTESIAN_POINT('Ctrl Pts',(-4.01183942564,-18.9153604797,-5.93052159234));
#98230=CARTESIAN_POINT('Ctrl Pts',(-3.98996412602,-18.9249461655,-5.99330285525));
#98231=CARTESIAN_POINT('Ctrl Pts',(-4.21445160765,-18.7590074427,-5.8013690143));
#98232=CARTESIAN_POINT('Ctrl Pts',(-4.14870486904,-18.782392944,-5.80464378088));
#98233=CARTESIAN_POINT('Ctrl Pts',(-4.08401276797,-18.8057784452,-5.82817429489));
#98234=CARTESIAN_POINT('Ctrl Pts',(-4.02780284558,-18.8265330161,-5.87164620833));
#98235=CARTESIAN_POINT('Ctrl Pts',(-3.98697746856,-18.8421086289,-5.92969706832));
#98236=CARTESIAN_POINT('Ctrl Pts',(-3.96404497635,-18.8514680746,-5.99493430976));
#98237=CARTESIAN_POINT('Ctrl Pts',(-4.2,-18.6809100188,-5.8013690143));
#98238=CARTESIAN_POINT('Ctrl Pts',(-4.1320193297,-18.7060691067,-5.8013690143));
#98239=CARTESIAN_POINT('Ctrl Pts',(-4.06403865941,-18.7312281946,-5.82326214445));
#98240=CARTESIAN_POINT('Ctrl Pts',(-4.00438514857,-18.7533054691,-5.8671585007));
#98241=CARTESIAN_POINT('Ctrl Pts',(-3.96107032516,-18.7693359296,-5.92716275717));
#98242=CARTESIAN_POINT('Ctrl Pts',(-3.9369519833,-18.7782619299,-5.99493430976));
#98243=CARTESIAN_POINT('',(-4.26546728923319,-19.0742356128,-5.79413859154276));
#98244=CARTESIAN_POINT('Ctrl Pts',(-4.2,-18.6809100188,-5.8013690143));
#98245=CARTESIAN_POINT('Ctrl Pts',(-4.22006430058665,-18.7893389122285,
-5.8013690143));
#98246=CARTESIAN_POINT('Ctrl Pts',(-4.23867827458747,-18.8984340287179,
-5.79935944419928));
#98247=CARTESIAN_POINT('Ctrl Pts',(-4.25554083761466,-19.0081708556049,
-5.79618275354226));
#98248=CARTESIAN_POINT('Ctrl Pts',(-4.2589207689943,-19.0301665002823,-5.79554601780892));
#98249=CARTESIAN_POINT('Ctrl Pts',(-4.2622303821849,-19.0521880859069,-5.79486234132898));
#98250=CARTESIAN_POINT('Ctrl Pts',(-4.26546727976036,-19.0742356128001,
-5.79413854918021));
#98251=CARTESIAN_POINT('Origin',(-4.33093462721,-19.0742356128,-6.08690818754));
#98252=CARTESIAN_POINT('Origin',(-4.33093462721,-19.0742356128,-6.08690818754));
#98253=CARTESIAN_POINT('Origin',(-4.33093462721,-19.0742356128,-6.08690818754));
#98254=CARTESIAN_POINT('Origin',(-4.2,-19.0742356128,-5.5013690143));
#98255=CARTESIAN_POINT('Origin',(-4.2,-19.0742356128,-5.5013690143));
#98256=CARTESIAN_POINT('Origin',(-4.2,-13.6742356128,-5.5013690143));
#98257=CARTESIAN_POINT('Origin',(0.,-16.6742356128,0.473661560394));
#98258=CARTESIAN_POINT('Origin',(-6.54794311523,-4.67423561284,3.49012794495));
#98259=CARTESIAN_POINT('',(-5.44794311523,-14.0742356128,3.49012794495));
#98260=CARTESIAN_POINT('',(-4.97448577881,-14.0742356128,3.49012794495));
#98261=CARTESIAN_POINT('',(-5.44794311523,-9.37423561284,3.49012794495));
#98262=CARTESIAN_POINT('Origin',(-5.44794311523,-4.67423561284,0.473661560394));
#98263=CARTESIAN_POINT('',(-5.44794311523,-14.0742356128,-2.54280482416));
#98264=CARTESIAN_POINT('',(-5.44794311523,-14.0742356128,1.98189475267));
#98265=CARTESIAN_POINT('',(-5.44794311523,-9.37423561284,-2.54280482416));
#98266=CARTESIAN_POINT('Origin',(0.,-14.0742356128,0.473661560394));
#98267=CARTESIAN_POINT('',(-4.97448577881,-14.0742356128,-2.54280482416));
#98268=CARTESIAN_POINT('Origin',(-6.54794311523,-4.67423561284,-2.54280482416));
#98289=UNCERTAINTY_MEASURE_WITH_UNIT(LENGTH_MEASURE(0.01),#98303,
'DISTANCE_ACCURACY_VALUE',
'Maximum model space distance between geometric entities at asserted c
onnectivities');
#98290=UNCERTAINTY_MEASURE_WITH_UNIT(LENGTH_MEASURE(0.01),#98303,
'DISTANCE_ACCURACY_VALUE',
'Maximum model space distance between geometric entities at asserted c
onnectivities');
#98301=(
GEOMETRIC_REPRESENTATION_CONTEXT(3)
GLOBAL_UNCERTAINTY_ASSIGNED_CONTEXT((#98289))
GLOBAL_UNIT_ASSIGNED_CONTEXT((#98303,#98305,#98306))
REPRESENTATION_CONTEXT('','3D')
);
#98302=(
GEOMETRIC_REPRESENTATION_CONTEXT(3)
GLOBAL_UNCERTAINTY_ASSIGNED_CONTEXT((#98290))
GLOBAL_UNIT_ASSIGNED_CONTEXT((#98303,#98305,#98306))
REPRESENTATION_CONTEXT('','3D')
);
#98303=(
LENGTH_UNIT()
NAMED_UNIT(*)
SI_UNIT(.MILLI.,.METRE.)
);
#98305=(
NAMED_UNIT(*)
PLANE_ANGLE_UNIT()
SI_UNIT($,.RADIAN.)
);
#98306=(
NAMED_UNIT(*)
SI_UNIT($,.STERADIAN.)
SOLID_ANGLE_UNIT()
);
#98317=SHAPE_DEFINITION_REPRESENTATION(#98328,#98349);
#98328=PRODUCT_DEFINITION_SHAPE('',$,#98361);
#98349=SHAPE_REPRESENTATION('',(#38347),#98301);
#98350=PRODUCT_DEFINITION_CONTEXT('part definition',#98385,'design');
#98361=PRODUCT_DEFINITION('Pivot Adapter','Pivot Adapter',#98372,#98350);
#98372=PRODUCT_DEFINITION_FORMATION('',$,#98397);
#98385=APPLICATION_CONTEXT(
'Core Data for Automotive Mechanical Design Process');
#98386=PRODUCT_CONTEXT('part definition',#98385,'mechanical');
#98397=PRODUCT('Pivot Adapter','Pivot Adapter',$,(#98386));
#98399=PRESENTATION_STYLE_ASSIGNMENT((#98401));
#98401=SURFACE_STYLE_USAGE(.BOTH.,#98403);
#98403=SURFACE_SIDE_STYLE('',(#98405));
#98405=SURFACE_STYLE_FILL_AREA(#98407);
#98407=FILL_AREA_STYLE('Opaque(202,209,238)',(#98409));
#98409=FILL_AREA_STYLE_COLOUR('Opaque(202,209,238)',#98411);
#98411=COLOUR_RGB('Opaque(202,209,238)', 0.31764706, 0.68627451, 0.89019608);
ENDSEC;
END-ISO-10303-21;
